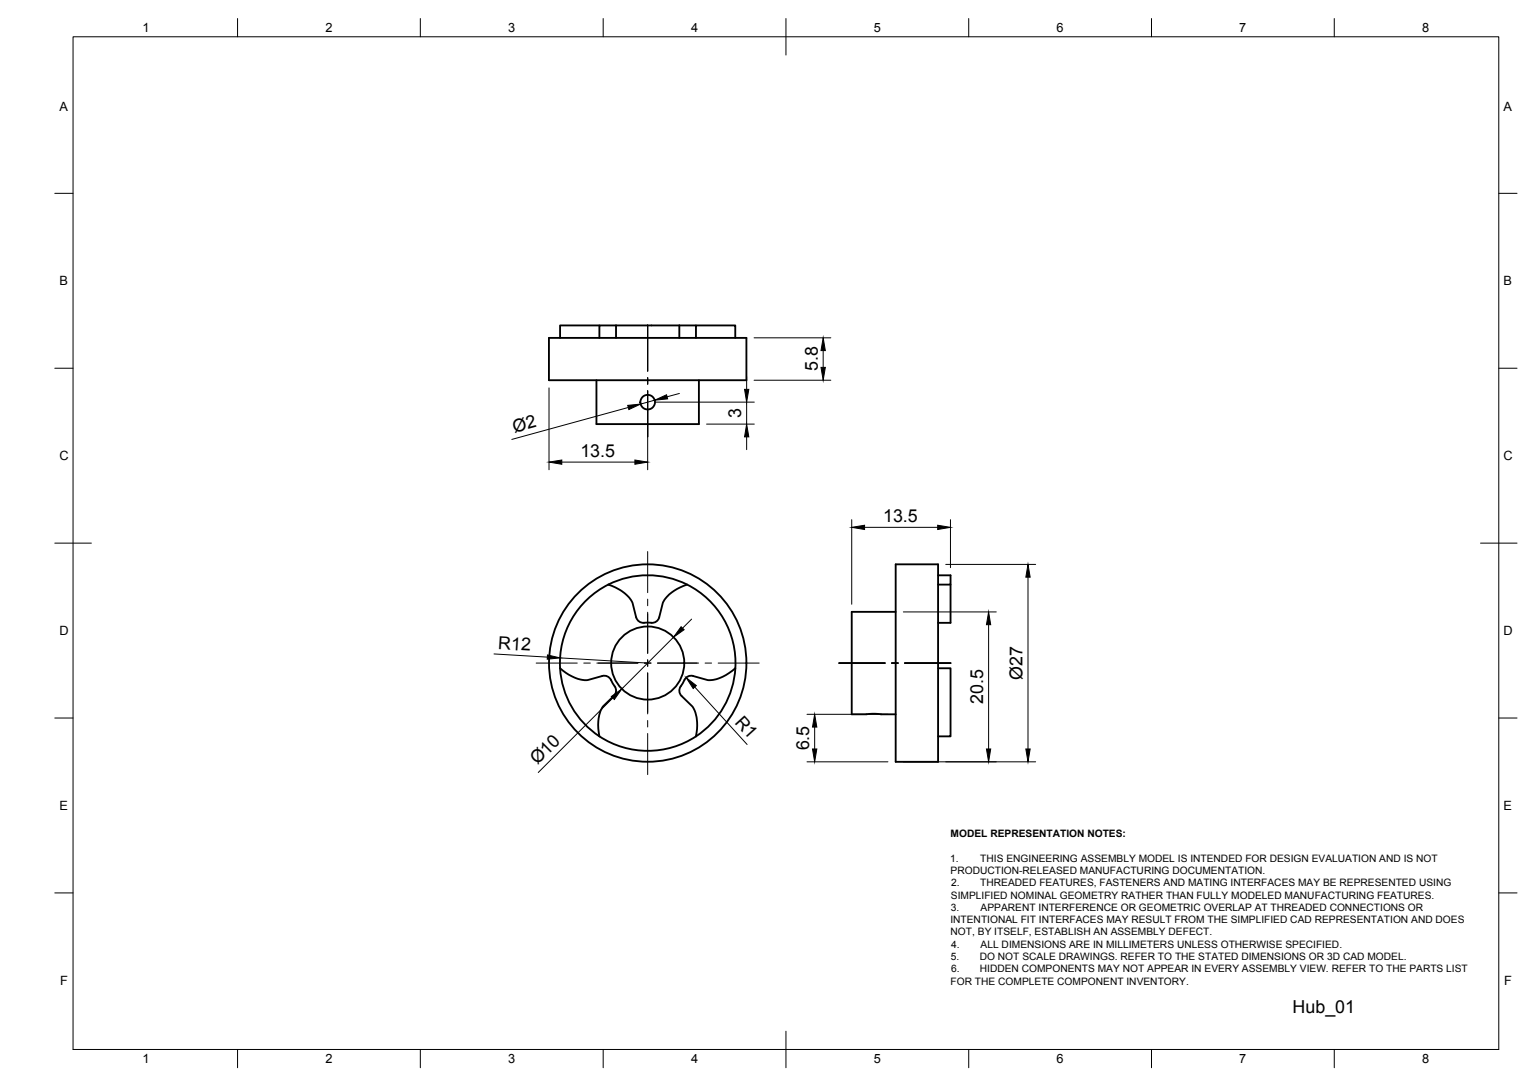
ISO-10303-21;
HEADER;
/* Generated by software containing ST-Developer
 * from STEP Tools, Inc. (www.steptools.com) 
 */

FILE_DESCRIPTION(
/* description */ (''),
/* implementation_level */ '2;1');

FILE_NAME(
/* name */ 'Hub_01.step',
/* time_stamp */ '2026-10-05T21:34:53-07:00',
/* author */ (''),
/* organization */ (''),
/* preprocessor_version */ 'ST-DEVELOPER v20.2',
/* originating_system */ 'Autodesk Translation Framework v15.15.0.0',
/* authorisation */ '');

FILE_SCHEMA (('AUTOMOTIVE_DESIGN { 1 0 10303 214 3 1 1 }'));
ENDSEC;

DATA;
#10=MECHANICAL_DESIGN_GEOMETRIC_PRESENTATION_REPRESENTATION('',(#66),#9822);
#48=SHAPE_REPRESENTATION_RELATIONSHIP('SRR','None',#9858,#57);
#57=ADVANCED_BREP_SHAPE_REPRESENTATION('',(#75),#9814);
#66=STYLED_ITEM('',(#9911),#75);
#75=MANIFOLD_SOLID_BREP('Body1',#3289);
#85=FACE_BOUND('',#514,.T.);
#86=FACE_BOUND('',#518,.T.);
#87=FACE_BOUND('',#520,.T.);
#88=FACE_BOUND('',#522,.T.);
#89=FACE_BOUND('',#525,.T.);
#123=B_SPLINE_CURVE_WITH_KNOTS('',3,(#8517,#8518,#8519,#8520,#8521,#8522,
#8523,#8524,#8525,#8526,#8527,#8528,#8529,#8530,#8531,#8532,#8533,#8534),
 .UNSPECIFIED.,.F.,.F.,(4,2,2,2,2,2,2,2,4),(0.,0.0377244205563716,0.0754488411127431,
0.113172721595804,0.150896602078865,0.188620482561925,0.226344363044986,
0.264068783601358,0.301793204157729),.UNSPECIFIED.);
#124=B_SPLINE_CURVE_WITH_KNOTS('',3,(#8535,#8536,#8537,#8538,#8539,#8540,
#8541,#8542,#8543,#8544,#8545,#8546,#8547,#8548,#8549,#8550,#8551,#8552),
 .UNSPECIFIED.,.F.,.F.,(4,2,2,2,2,2,2,2,4),(0.301793204157729,0.339517624714101,
0.377242045270472,0.414965925753533,0.452689806236594,0.490413686719655,
0.528137567202715,0.565861987759087,0.603586408315459),.UNSPECIFIED.);
#125=B_SPLINE_CURVE_WITH_KNOTS('',3,(#8568,#8569,#8570,#8571,#8572,#8573,
#8574,#8575,#8576,#8577,#8578,#8579,#8580,#8581,#8582,#8583,#8584,#8585),
 .UNSPECIFIED.,.F.,.F.,(4,2,2,2,2,2,2,2,4),(-0.302227736861757,-0.264448211272738,
-0.226668685683718,-0.188891277057298,-0.151113868430879,-0.113336459804459,
-0.0755590511780388,-0.0377795255890194,0.),.UNSPECIFIED.);
#126=B_SPLINE_CURVE_WITH_KNOTS('',3,(#8650,#8651,#8652,#8653,#8654,#8655,
#8656,#8657,#8658,#8659),.UNSPECIFIED.,.F.,.F.,(4,2,2,2,4),(-1.69587030996743,
-0.72373117051105,-0.441822634822492,-0.252830368895713,0.),
 .UNSPECIFIED.);
#127=B_SPLINE_CURVE_WITH_KNOTS('',3,(#8670,#8671,#8672,#8673,#8674,#8675,
#8676,#8677,#8678,#8679),.UNSPECIFIED.,.F.,.F.,(4,2,2,2,4),(-0.142515337540036,
-0.116550796137795,-0.0827833358078941,-0.0239794870259568,0.),
 .UNSPECIFIED.);
#128=B_SPLINE_CURVE_WITH_KNOTS('',3,(#8681,#8682,#8683,#8684,#8685,#8686,
#8687,#8688,#8689,#8690),.UNSPECIFIED.,.F.,.F.,(4,2,2,2,4),(-1.69587031141743,
-0.723731170975569,-0.441822635061051,-0.252830368989318,0.),
 .UNSPECIFIED.);
#129=B_SPLINE_CURVE_WITH_KNOTS('',3,(#8701,#8702,#8703,#8704,#8705,#8706,
#8707,#8708,#8709,#8710),.UNSPECIFIED.,.F.,.F.,(4,2,2,2,4),(-0.142515337583282,
-0.116550796158019,-0.0827833358058086,-0.0239794870257561,0.),
 .UNSPECIFIED.);
#130=B_SPLINE_CURVE_WITH_KNOTS('',3,(#8712,#8713,#8714,#8715,#8716,#8717,
#8718,#8719,#8720,#8721),.UNSPECIFIED.,.F.,.F.,(4,2,2,2,4),(-1.69587031053129,
-0.72373117069956,-0.441822634924292,-0.252830368936358,0.),
 .UNSPECIFIED.);
#131=B_SPLINE_CURVE_WITH_KNOTS('',3,(#8732,#8733,#8734,#8735,#8736,#8737,
#8738,#8739,#8740,#8741),.UNSPECIFIED.,.F.,.F.,(4,2,2,2,4),(-0.142515337525874,
-0.116550796129695,-0.0827833358062311,-0.0239794870259187,0.),
 .UNSPECIFIED.);
#132=B_SPLINE_CURVE_WITH_KNOTS('',3,(#8788,#8789,#8790,#8791,#8792,#8793,
#8794,#8795,#8796,#8797),.UNSPECIFIED.,.F.,.F.,(4,2,2,2,4),(-0.142515337540036,
-0.116550796137795,-0.0827833358078941,-0.0239794870259568,0.),
 .UNSPECIFIED.);
#133=B_SPLINE_CURVE_WITH_KNOTS('',3,(#8819,#8820,#8821,#8822,#8823,#8824,
#8825,#8826,#8827,#8828),.UNSPECIFIED.,.F.,.F.,(4,2,2,2,4),(-1.69587030996743,
-0.72373117051105,-0.441822634822492,-0.252830368895713,0.),
 .UNSPECIFIED.);
#134=B_SPLINE_CURVE_WITH_KNOTS('',3,(#8871,#8872,#8873,#8874,#8875,#8876,
#8877,#8878,#8879,#8880),.UNSPECIFIED.,.F.,.F.,(4,2,2,2,4),(-0.142515337583282,
-0.116550796158019,-0.0827833358058086,-0.0239794870257561,0.),
 .UNSPECIFIED.);
#135=B_SPLINE_CURVE_WITH_KNOTS('',3,(#8902,#8903,#8904,#8905,#8906,#8907,
#8908,#8909,#8910,#8911),.UNSPECIFIED.,.F.,.F.,(4,2,2,2,4),(-1.69587031141743,
-0.723731170975569,-0.441822635061051,-0.252830368989318,0.),
 .UNSPECIFIED.);
#136=B_SPLINE_CURVE_WITH_KNOTS('',3,(#8955,#8956,#8957,#8958,#8959,#8960,
#8961,#8962,#8963,#8964),.UNSPECIFIED.,.F.,.F.,(4,2,2,2,4),(-0.142515337525874,
-0.116550796129695,-0.0827833358062311,-0.0239794870259187,0.),
 .UNSPECIFIED.);
#137=B_SPLINE_CURVE_WITH_KNOTS('',3,(#8991,#8992,#8993,#8994,#8995,#8996,
#8997,#8998,#8999,#9000),.UNSPECIFIED.,.F.,.F.,(4,2,2,2,4),(-1.69587031053129,
-0.72373117069956,-0.441822634924292,-0.252830368936358,0.),
 .UNSPECIFIED.);
#169=B_SPLINE_SURFACE_WITH_KNOTS('',3,1,((#8768,#8769),(#8770,#8771),(#8772,
#8773),(#8774,#8775),(#8776,#8777),(#8778,#8779),(#8780,#8781),(#8782,#8783),
(#8784,#8785),(#8786,#8787)),.UNSPECIFIED.,.F.,.F.,.F.,(4,2,2,2,4),(2,2),
(-0.142515337540036,-0.116550796137795,-0.0827833358078941,-0.0239794870259568,
0.),(0.,0.78),.UNSPECIFIED.);
#170=B_SPLINE_SURFACE_WITH_KNOTS('',3,1,((#8798,#8799),(#8800,#8801),(#8802,
#8803),(#8804,#8805),(#8806,#8807),(#8808,#8809),(#8810,#8811),(#8812,#8813),
(#8814,#8815),(#8816,#8817)),.UNSPECIFIED.,.F.,.F.,.F.,(4,2,2,2,4),(2,2),
(-1.69587030996743,-0.72373117051105,-0.441822634822492,-0.252830368895713,
0.),(0.,0.78),.UNSPECIFIED.);
#171=B_SPLINE_SURFACE_WITH_KNOTS('',3,1,((#8851,#8852),(#8853,#8854),(#8855,
#8856),(#8857,#8858),(#8859,#8860),(#8861,#8862),(#8863,#8864),(#8865,#8866),
(#8867,#8868),(#8869,#8870)),.UNSPECIFIED.,.F.,.F.,.F.,(4,2,2,2,4),(2,2),
(-0.142515337583282,-0.116550796158019,-0.0827833358058086,-0.0239794870257561,
0.),(0.,0.78),.UNSPECIFIED.);
#172=B_SPLINE_SURFACE_WITH_KNOTS('',3,1,((#8881,#8882),(#8883,#8884),(#8885,
#8886),(#8887,#8888),(#8889,#8890),(#8891,#8892),(#8893,#8894),(#8895,#8896),
(#8897,#8898),(#8899,#8900)),.UNSPECIFIED.,.F.,.F.,.F.,(4,2,2,2,4),(2,2),
(-1.69587031141743,-0.723731170975569,-0.441822635061051,-0.252830368989318,
0.),(0.,0.78),.UNSPECIFIED.);
#173=B_SPLINE_SURFACE_WITH_KNOTS('',3,1,((#8934,#8935),(#8936,#8937),(#8938,
#8939),(#8940,#8941),(#8942,#8943),(#8944,#8945),(#8946,#8947),(#8948,#8949),
(#8950,#8951),(#8952,#8953)),.UNSPECIFIED.,.F.,.F.,.F.,(4,2,2,2,4),(2,2),
(-0.142515337525874,-0.116550796129695,-0.0827833358062311,-0.0239794870259187,
0.),(0.,0.78),.UNSPECIFIED.);
#174=B_SPLINE_SURFACE_WITH_KNOTS('',3,1,((#8970,#8971),(#8972,#8973),(#8974,
#8975),(#8976,#8977),(#8978,#8979),(#8980,#8981),(#8982,#8983),(#8984,#8985),
(#8986,#8987),(#8988,#8989)),.UNSPECIFIED.,.F.,.F.,.F.,(4,2,2,2,4),(2,2),
(-1.69587031053129,-0.72373117069956,-0.441822634924292,-0.252830368936358,
0.),(0.,0.78),.UNSPECIFIED.);
#195=PLANE('',#3492);
#196=PLANE('',#3494);
#197=PLANE('',#3496);
#198=PLANE('',#3497);
#199=PLANE('',#3511);
#200=PLANE('',#3520);
#201=PLANE('',#3533);
#202=PLANE('',#3536);
#203=PLANE('',#3541);
#204=PLANE('',#3542);
#205=PLANE('',#3545);
#206=PLANE('',#3550);
#207=PLANE('',#3551);
#208=PLANE('',#3554);
#209=PLANE('',#3559);
#210=PLANE('',#3562);
#211=PLANE('',#3565);
#316=FACE_OUTER_BOUND('',#503,.T.);
#317=FACE_OUTER_BOUND('',#504,.T.);
#318=FACE_OUTER_BOUND('',#505,.T.);
#319=FACE_OUTER_BOUND('',#506,.T.);
#320=FACE_OUTER_BOUND('',#507,.T.);
#321=FACE_OUTER_BOUND('',#508,.T.);
#322=FACE_OUTER_BOUND('',#509,.T.);
#323=FACE_OUTER_BOUND('',#510,.T.);
#324=FACE_OUTER_BOUND('',#511,.T.);
#325=FACE_OUTER_BOUND('',#512,.T.);
#326=FACE_OUTER_BOUND('',#513,.T.);
#327=FACE_OUTER_BOUND('',#515,.T.);
#328=FACE_OUTER_BOUND('',#516,.T.);
#329=FACE_OUTER_BOUND('',#517,.T.);
#330=FACE_OUTER_BOUND('',#519,.T.);
#331=FACE_OUTER_BOUND('',#521,.T.);
#332=FACE_OUTER_BOUND('',#523,.T.);
#333=FACE_OUTER_BOUND('',#524,.T.);
#334=FACE_OUTER_BOUND('',#526,.T.);
#335=FACE_OUTER_BOUND('',#527,.T.);
#336=FACE_OUTER_BOUND('',#528,.T.);
#337=FACE_OUTER_BOUND('',#529,.T.);
#338=FACE_OUTER_BOUND('',#530,.T.);
#339=FACE_OUTER_BOUND('',#531,.T.);
#340=FACE_OUTER_BOUND('',#532,.T.);
#341=FACE_OUTER_BOUND('',#533,.T.);
#342=FACE_OUTER_BOUND('',#534,.T.);
#343=FACE_OUTER_BOUND('',#535,.T.);
#344=FACE_OUTER_BOUND('',#536,.T.);
#345=FACE_OUTER_BOUND('',#537,.T.);
#346=FACE_OUTER_BOUND('',#538,.T.);
#347=FACE_OUTER_BOUND('',#539,.T.);
#348=FACE_OUTER_BOUND('',#540,.T.);
#349=FACE_OUTER_BOUND('',#541,.T.);
#350=FACE_OUTER_BOUND('',#542,.T.);
#351=FACE_OUTER_BOUND('',#543,.T.);
#352=FACE_OUTER_BOUND('',#544,.T.);
#353=FACE_OUTER_BOUND('',#545,.T.);
#354=FACE_OUTER_BOUND('',#546,.T.);
#355=FACE_OUTER_BOUND('',#547,.T.);
#356=FACE_OUTER_BOUND('',#548,.T.);
#357=FACE_OUTER_BOUND('',#549,.T.);
#358=FACE_OUTER_BOUND('',#550,.T.);
#503=EDGE_LOOP('',(#2386,#2387,#2388,#2389,#2390,#2391));
#504=EDGE_LOOP('',(#2392,#2393,#2394,#2395));
#505=EDGE_LOOP('',(#2396,#2397,#2398,#2399));
#506=EDGE_LOOP('',(#2400,#2401,#2402,#2403));
#507=EDGE_LOOP('',(#2404,#2405,#2406,#2407,#2408));
#508=EDGE_LOOP('',(#2409,#2410,#2411,#2412,#2413));
#509=EDGE_LOOP('',(#2414,#2415,#2416,#2417,#2418,#2419,#2420,#2421));
#510=EDGE_LOOP('',(#2422,#2423,#2424,#2425));
#511=EDGE_LOOP('',(#2426,#2427,#2428,#2429));
#512=EDGE_LOOP('',(#2430,#2431,#2432,#2433));
#513=EDGE_LOOP('',(#2434));
#514=EDGE_LOOP('',(#2435,#2436,#2437,#2438,#2439,#2440));
#515=EDGE_LOOP('',(#2441,#2442,#2443,#2444));
#516=EDGE_LOOP('',(#2445,#2446,#2447,#2448));
#517=EDGE_LOOP('',(#2449,#2450,#2451,#2452,#2453,#2454,#2455,#2456,#2457,
#2458,#2459,#2460,#2461,#2462,#2463,#2464,#2465,#2466,#2467,#2468,#2469,
#2470,#2471,#2472));
#518=EDGE_LOOP('',(#2473));
#519=EDGE_LOOP('',(#2474,#2475,#2476,#2477));
#520=EDGE_LOOP('',(#2478,#2479));
#521=EDGE_LOOP('',(#2480));
#522=EDGE_LOOP('',(#2481,#2482,#2483,#2484,#2485));
#523=EDGE_LOOP('',(#2486,#2487,#2488,#2489));
#524=EDGE_LOOP('',(#2490));
#525=EDGE_LOOP('',(#2491));
#526=EDGE_LOOP('',(#2492,#2493,#2494,#2495));
#527=EDGE_LOOP('',(#2496,#2497,#2498,#2499));
#528=EDGE_LOOP('',(#2500,#2501,#2502,#2503));
#529=EDGE_LOOP('',(#2504,#2505,#2506,#2507,#2508));
#530=EDGE_LOOP('',(#2509,#2510,#2511,#2512,#2513));
#531=EDGE_LOOP('',(#2514,#2515,#2516,#2517));
#532=EDGE_LOOP('',(#2518,#2519,#2520,#2521));
#533=EDGE_LOOP('',(#2522,#2523,#2524,#2525,#2526,#2527,#2528,#2529));
#534=EDGE_LOOP('',(#2530,#2531,#2532,#2533));
#535=EDGE_LOOP('',(#2534,#2535,#2536,#2537));
#536=EDGE_LOOP('',(#2538,#2539,#2540,#2541));
#537=EDGE_LOOP('',(#2542,#2543,#2544,#2545,#2546));
#538=EDGE_LOOP('',(#2547,#2548,#2549,#2550,#2551));
#539=EDGE_LOOP('',(#2552,#2553,#2554,#2555));
#540=EDGE_LOOP('',(#2556,#2557,#2558,#2559));
#541=EDGE_LOOP('',(#2560,#2561,#2562,#2563,#2564,#2565,#2566,#2567));
#542=EDGE_LOOP('',(#2568,#2569,#2570,#2571));
#543=EDGE_LOOP('',(#2572,#2573,#2574,#2575));
#544=EDGE_LOOP('',(#2576,#2577,#2578,#2579));
#545=EDGE_LOOP('',(#2580,#2581,#2582,#2583,#2584));
#546=EDGE_LOOP('',(#2585,#2586,#2587,#2588));
#547=EDGE_LOOP('',(#2589,#2590,#2591,#2592,#2593));
#548=EDGE_LOOP('',(#2594,#2595,#2596,#2597));
#549=EDGE_LOOP('',(#2598,#2599,#2600,#2601));
#550=EDGE_LOOP('',(#2602,#2603,#2604,#2605,#2606,#2607,#2608,#2609));
#724=LINE('',#8515,#983);
#725=LINE('',#8555,#984);
#726=LINE('',#8558,#985);
#727=LINE('',#8561,#986);
#728=LINE('',#8563,#987);
#729=LINE('',#8564,#988);
#730=LINE('',#8586,#989);
#731=LINE('',#8587,#990);
#732=LINE('',#8590,#991);
#733=LINE('',#8591,#992);
#734=LINE('',#8594,#993);
#735=LINE('',#8595,#994);
#736=LINE('',#8600,#995);
#737=LINE('',#8606,#996);
#738=LINE('',#8610,#997);
#739=LINE('',#8615,#998);
#740=LINE('',#8619,#999);
#741=LINE('',#8624,#1000);
#742=LINE('',#8628,#1001);
#743=LINE('',#8638,#1002);
#744=LINE('',#8641,#1003);
#745=LINE('',#8644,#1004);
#746=LINE('',#8647,#1005);
#747=LINE('',#8661,#1006);
#748=LINE('',#8669,#1007);
#749=LINE('',#8692,#1008);
#750=LINE('',#8700,#1009);
#751=LINE('',#8723,#1010);
#752=LINE('',#8731,#1011);
#753=LINE('',#8746,#1012);
#754=LINE('',#8752,#1013);
#755=LINE('',#8756,#1014);
#756=LINE('',#8759,#1015);
#757=LINE('',#8763,#1016);
#758=LINE('',#8766,#1017);
#759=LINE('',#8767,#1018);
#760=LINE('',#8829,#1019);
#761=LINE('',#8832,#1020);
#762=LINE('',#8833,#1021);
#763=LINE('',#8839,#1022);
#764=LINE('',#8842,#1023);
#765=LINE('',#8846,#1024);
#766=LINE('',#8849,#1025);
#767=LINE('',#8850,#1026);
#768=LINE('',#8912,#1027);
#769=LINE('',#8915,#1028);
#770=LINE('',#8916,#1029);
#771=LINE('',#8922,#1030);
#772=LINE('',#8925,#1031);
#773=LINE('',#8929,#1032);
#774=LINE('',#8932,#1033);
#775=LINE('',#8933,#1034);
#776=LINE('',#8965,#1035);
#777=LINE('',#8969,#1036);
#778=LINE('',#9001,#1037);
#779=LINE('',#9004,#1038);
#780=LINE('',#9005,#1039);
#983=VECTOR('',#3990,1.);
#984=VECTOR('',#3993,10.);
#985=VECTOR('',#3996,10.);
#986=VECTOR('',#3999,10.);
#987=VECTOR('',#4000,10.);
#988=VECTOR('',#4001,10.);
#989=VECTOR('',#4004,10.);
#990=VECTOR('',#4005,10.);
#991=VECTOR('',#4008,10.);
#992=VECTOR('',#4009,10.);
#993=VECTOR('',#4012,10.);
#994=VECTOR('',#4013,10.);
#995=VECTOR('',#4018,5.);
#996=VECTOR('',#4025,10.);
#997=VECTOR('',#4028,10.);
#998=VECTOR('',#4033,10.);
#999=VECTOR('',#4036,10.);
#1000=VECTOR('',#4041,10.);
#1001=VECTOR('',#4044,10.);
#1002=VECTOR('',#4059,10.);
#1003=VECTOR('',#4062,10.);
#1004=VECTOR('',#4065,10.);
#1005=VECTOR('',#4068,10.);
#1006=VECTOR('',#4071,10.);
#1007=VECTOR('',#4078,10.);
#1008=VECTOR('',#4079,10.);
#1009=VECTOR('',#4086,10.);
#1010=VECTOR('',#4087,10.);
#1011=VECTOR('',#4094,10.);
#1012=VECTOR('',#4099,7.);
#1013=VECTOR('',#4108,13.5);
#1014=VECTOR('',#4113,10.);
#1015=VECTOR('',#4116,10.);
#1016=VECTOR('',#4121,10.);
#1017=VECTOR('',#4124,10.);
#1018=VECTOR('',#4125,10.);
#1019=VECTOR('',#4126,10.);
#1020=VECTOR('',#4129,10.);
#1021=VECTOR('',#4130,10.);
#1022=VECTOR('',#4139,10.);
#1023=VECTOR('',#4142,10.);
#1024=VECTOR('',#4147,10.);
#1025=VECTOR('',#4150,10.);
#1026=VECTOR('',#4151,10.);
#1027=VECTOR('',#4152,10.);
#1028=VECTOR('',#4155,10.);
#1029=VECTOR('',#4156,10.);
#1030=VECTOR('',#4165,10.);
#1031=VECTOR('',#4168,10.);
#1032=VECTOR('',#4173,10.);
#1033=VECTOR('',#4176,10.);
#1034=VECTOR('',#4177,10.);
#1035=VECTOR('',#4178,10.);
#1036=VECTOR('',#4183,10.);
#1037=VECTOR('',#4184,10.);
#1038=VECTOR('',#4187,10.);
#1039=VECTOR('',#4188,10.);
#1219=CIRCLE('',#3490,1.);
#1220=CIRCLE('',#3491,1.);
#1221=CIRCLE('',#3493,1.);
#1222=CIRCLE('',#3499,5.);
#1223=CIRCLE('',#3500,5.);
#1224=CIRCLE('',#3501,5.);
#1225=CIRCLE('',#3503,12.);
#1226=CIRCLE('',#3504,12.);
#1227=CIRCLE('',#3506,12.);
#1228=CIRCLE('',#3507,12.);
#1229=CIRCLE('',#3509,12.);
#1230=CIRCLE('',#3510,12.);
#1231=CIRCLE('',#3512,13.5);
#1232=CIRCLE('',#3513,12.);
#1233=CIRCLE('',#3514,12.);
#1234=CIRCLE('',#3515,12.);
#1235=CIRCLE('',#3517,12.);
#1236=CIRCLE('',#3519,12.);
#1237=CIRCLE('',#3521,1.);
#1238=CIRCLE('',#3522,5.529);
#1239=CIRCLE('',#3523,1.);
#1240=CIRCLE('',#3524,1.);
#1241=CIRCLE('',#3525,5.529);
#1242=CIRCLE('',#3526,1.);
#1243=CIRCLE('',#3527,1.);
#1244=CIRCLE('',#3528,5.529);
#1245=CIRCLE('',#3529,1.);
#1246=CIRCLE('',#3531,7.);
#1247=CIRCLE('',#3532,7.);
#1248=CIRCLE('',#3535,13.5);
#1249=CIRCLE('',#3538,5.529);
#1250=CIRCLE('',#3540,1.);
#1251=CIRCLE('',#3544,1.);
#1252=CIRCLE('',#3547,5.529);
#1253=CIRCLE('',#3549,1.);
#1254=CIRCLE('',#3553,1.);
#1255=CIRCLE('',#3556,5.529);
#1256=CIRCLE('',#3558,1.);
#1257=CIRCLE('',#3561,12.);
#1258=CIRCLE('',#3564,1.);
#1417=VERTEX_POINT('',#8510);
#1418=VERTEX_POINT('',#8511);
#1419=VERTEX_POINT('',#8514);
#1420=VERTEX_POINT('',#8516);
#1421=VERTEX_POINT('',#8554);
#1422=VERTEX_POINT('',#8556);
#1423=VERTEX_POINT('',#8560);
#1424=VERTEX_POINT('',#8562);
#1425=VERTEX_POINT('',#8566);
#1426=VERTEX_POINT('',#8567);
#1427=VERTEX_POINT('',#8589);
#1428=VERTEX_POINT('',#8593);
#1429=VERTEX_POINT('',#8597);
#1430=VERTEX_POINT('',#8599);
#1431=VERTEX_POINT('',#8604);
#1432=VERTEX_POINT('',#8605);
#1433=VERTEX_POINT('',#8607);
#1434=VERTEX_POINT('',#8609);
#1435=VERTEX_POINT('',#8613);
#1436=VERTEX_POINT('',#8614);
#1437=VERTEX_POINT('',#8616);
#1438=VERTEX_POINT('',#8618);
#1439=VERTEX_POINT('',#8622);
#1440=VERTEX_POINT('',#8623);
#1441=VERTEX_POINT('',#8625);
#1442=VERTEX_POINT('',#8627);
#1443=VERTEX_POINT('',#8631);
#1444=VERTEX_POINT('',#8637);
#1445=VERTEX_POINT('',#8639);
#1446=VERTEX_POINT('',#8643);
#1447=VERTEX_POINT('',#8645);
#1448=VERTEX_POINT('',#8649);
#1449=VERTEX_POINT('',#8660);
#1450=VERTEX_POINT('',#8662);
#1451=VERTEX_POINT('',#8664);
#1452=VERTEX_POINT('',#8666);
#1453=VERTEX_POINT('',#8668);
#1454=VERTEX_POINT('',#8680);
#1455=VERTEX_POINT('',#8691);
#1456=VERTEX_POINT('',#8693);
#1457=VERTEX_POINT('',#8695);
#1458=VERTEX_POINT('',#8697);
#1459=VERTEX_POINT('',#8699);
#1460=VERTEX_POINT('',#8711);
#1461=VERTEX_POINT('',#8722);
#1462=VERTEX_POINT('',#8724);
#1463=VERTEX_POINT('',#8726);
#1464=VERTEX_POINT('',#8728);
#1465=VERTEX_POINT('',#8730);
#1466=VERTEX_POINT('',#8743);
#1467=VERTEX_POINT('',#8745);
#1468=VERTEX_POINT('',#8750);
#1469=VERTEX_POINT('',#8755);
#1470=VERTEX_POINT('',#8757);
#1471=VERTEX_POINT('',#8761);
#1472=VERTEX_POINT('',#8765);
#1473=VERTEX_POINT('',#8818);
#1474=VERTEX_POINT('',#8831);
#1475=VERTEX_POINT('',#8838);
#1476=VERTEX_POINT('',#8840);
#1477=VERTEX_POINT('',#8844);
#1478=VERTEX_POINT('',#8848);
#1479=VERTEX_POINT('',#8901);
#1480=VERTEX_POINT('',#8914);
#1481=VERTEX_POINT('',#8921);
#1482=VERTEX_POINT('',#8923);
#1483=VERTEX_POINT('',#8927);
#1484=VERTEX_POINT('',#8931);
#1485=VERTEX_POINT('',#8954);
#1486=VERTEX_POINT('',#8967);
#1487=VERTEX_POINT('',#8990);
#1488=VERTEX_POINT('',#9003);
#1772=EDGE_CURVE('',#1417,#1418,#1219,.T.);
#1773=EDGE_CURVE('',#1418,#1417,#1220,.T.);
#1774=EDGE_CURVE('',#1418,#1419,#724,.T.);
#1775=EDGE_CURVE('',#1420,#1419,#123,.T.);
#1776=EDGE_CURVE('',#1419,#1420,#124,.T.);
#1777=EDGE_CURVE('',#1421,#1417,#725,.T.);
#1778=EDGE_CURVE('',#1422,#1421,#1221,.T.);
#1779=EDGE_CURVE('',#1418,#1422,#726,.T.);
#1780=EDGE_CURVE('',#1423,#1418,#727,.T.);
#1781=EDGE_CURVE('',#1424,#1423,#728,.T.);
#1782=EDGE_CURVE('',#1417,#1424,#729,.T.);
#1783=EDGE_CURVE('',#1425,#1426,#125,.T.);
#1784=EDGE_CURVE('',#1425,#1422,#730,.T.);
#1785=EDGE_CURVE('',#1426,#1421,#731,.T.);
#1786=EDGE_CURVE('',#1426,#1427,#732,.T.);
#1787=EDGE_CURVE('',#1427,#1424,#733,.T.);
#1788=EDGE_CURVE('',#1428,#1425,#734,.T.);
#1789=EDGE_CURVE('',#1423,#1428,#735,.T.);
#1790=EDGE_CURVE('',#1429,#1429,#1222,.T.);
#1791=EDGE_CURVE('',#1429,#1430,#736,.T.);
#1792=EDGE_CURVE('',#1428,#1430,#1223,.T.);
#1793=EDGE_CURVE('',#1430,#1427,#1224,.T.);
#1794=EDGE_CURVE('',#1431,#1432,#737,.T.);
#1795=EDGE_CURVE('',#1433,#1431,#1225,.T.);
#1796=EDGE_CURVE('',#1433,#1434,#738,.T.);
#1797=EDGE_CURVE('',#1432,#1434,#1226,.T.);
#1798=EDGE_CURVE('',#1435,#1436,#739,.T.);
#1799=EDGE_CURVE('',#1437,#1436,#1227,.T.);
#1800=EDGE_CURVE('',#1438,#1437,#740,.T.);
#1801=EDGE_CURVE('',#1435,#1438,#1228,.T.);
#1802=EDGE_CURVE('',#1439,#1440,#741,.T.);
#1803=EDGE_CURVE('',#1441,#1440,#1229,.T.);
#1804=EDGE_CURVE('',#1442,#1441,#742,.T.);
#1805=EDGE_CURVE('',#1439,#1442,#1230,.T.);
#1806=EDGE_CURVE('',#1443,#1443,#1231,.T.);
#1807=EDGE_CURVE('',#1441,#1436,#1232,.T.);
#1808=EDGE_CURVE('',#1432,#1440,#1233,.T.);
#1809=EDGE_CURVE('',#1437,#1434,#1234,.T.);
#1810=EDGE_CURVE('',#1436,#1444,#743,.T.);
#1811=EDGE_CURVE('',#1445,#1444,#1235,.T.);
#1812=EDGE_CURVE('',#1441,#1445,#744,.T.);
#1813=EDGE_CURVE('',#1434,#1446,#745,.T.);
#1814=EDGE_CURVE('',#1447,#1446,#1236,.T.);
#1815=EDGE_CURVE('',#1437,#1447,#746,.T.);
#1816=EDGE_CURVE('',#1448,#1442,#126,.T.);
#1817=EDGE_CURVE('',#1449,#1448,#747,.T.);
#1818=EDGE_CURVE('',#1449,#1450,#1237,.T.);
#1819=EDGE_CURVE('',#1451,#1450,#1238,.T.);
#1820=EDGE_CURVE('',#1451,#1452,#1239,.T.);
#1821=EDGE_CURVE('',#1453,#1452,#748,.T.);
#1822=EDGE_CURVE('',#1435,#1453,#127,.T.);
#1823=EDGE_CURVE('',#1454,#1438,#128,.T.);
#1824=EDGE_CURVE('',#1455,#1454,#749,.T.);
#1825=EDGE_CURVE('',#1455,#1456,#1240,.T.);
#1826=EDGE_CURVE('',#1457,#1456,#1241,.T.);
#1827=EDGE_CURVE('',#1457,#1458,#1242,.T.);
#1828=EDGE_CURVE('',#1459,#1458,#750,.T.);
#1829=EDGE_CURVE('',#1433,#1459,#129,.T.);
#1830=EDGE_CURVE('',#1460,#1431,#130,.T.);
#1831=EDGE_CURVE('',#1461,#1460,#751,.T.);
#1832=EDGE_CURVE('',#1461,#1462,#1243,.T.);
#1833=EDGE_CURVE('',#1463,#1462,#1244,.T.);
#1834=EDGE_CURVE('',#1463,#1464,#1245,.T.);
#1835=EDGE_CURVE('',#1465,#1464,#752,.T.);
#1836=EDGE_CURVE('',#1439,#1465,#131,.T.);
#1837=EDGE_CURVE('',#1466,#1466,#1246,.F.);
#1838=EDGE_CURVE('',#1466,#1467,#753,.T.);
#1839=EDGE_CURVE('',#1467,#1467,#1247,.T.);
#1840=EDGE_CURVE('',#1468,#1468,#1248,.T.);
#1841=EDGE_CURVE('',#1468,#1443,#754,.T.);
#1842=EDGE_CURVE('',#1450,#1469,#755,.T.);
#1843=EDGE_CURVE('',#1470,#1469,#1249,.T.);
#1844=EDGE_CURVE('',#1451,#1470,#756,.T.);
#1845=EDGE_CURVE('',#1471,#1470,#1250,.T.);
#1846=EDGE_CURVE('',#1452,#1471,#757,.T.);
#1847=EDGE_CURVE('',#1472,#1471,#758,.T.);
#1848=EDGE_CURVE('',#1453,#1472,#759,.T.);
#1849=EDGE_CURVE('',#1444,#1472,#132,.T.);
#1850=EDGE_CURVE('',#1473,#1445,#133,.T.);
#1851=EDGE_CURVE('',#1448,#1473,#760,.T.);
#1852=EDGE_CURVE('',#1474,#1473,#761,.T.);
#1853=EDGE_CURVE('',#1449,#1474,#762,.T.);
#1854=EDGE_CURVE('',#1469,#1474,#1251,.T.);
#1855=EDGE_CURVE('',#1456,#1475,#763,.T.);
#1856=EDGE_CURVE('',#1476,#1475,#1252,.T.);
#1857=EDGE_CURVE('',#1457,#1476,#764,.T.);
#1858=EDGE_CURVE('',#1477,#1476,#1253,.T.);
#1859=EDGE_CURVE('',#1458,#1477,#765,.T.);
#1860=EDGE_CURVE('',#1478,#1477,#766,.T.);
#1861=EDGE_CURVE('',#1459,#1478,#767,.T.);
#1862=EDGE_CURVE('',#1446,#1478,#134,.T.);
#1863=EDGE_CURVE('',#1479,#1447,#135,.T.);
#1864=EDGE_CURVE('',#1454,#1479,#768,.T.);
#1865=EDGE_CURVE('',#1480,#1479,#769,.T.);
#1866=EDGE_CURVE('',#1455,#1480,#770,.T.);
#1867=EDGE_CURVE('',#1475,#1480,#1254,.T.);
#1868=EDGE_CURVE('',#1462,#1481,#771,.T.);
#1869=EDGE_CURVE('',#1482,#1481,#1255,.T.);
#1870=EDGE_CURVE('',#1463,#1482,#772,.T.);
#1871=EDGE_CURVE('',#1483,#1482,#1256,.T.);
#1872=EDGE_CURVE('',#1464,#1483,#773,.T.);
#1873=EDGE_CURVE('',#1484,#1483,#774,.T.);
#1874=EDGE_CURVE('',#1465,#1484,#775,.T.);
#1875=EDGE_CURVE('',#1485,#1484,#136,.T.);
#1876=EDGE_CURVE('',#1440,#1485,#776,.T.);
#1877=EDGE_CURVE('',#1486,#1485,#1257,.T.);
#1878=EDGE_CURVE('',#1432,#1486,#777,.T.);
#1879=EDGE_CURVE('',#1487,#1486,#137,.T.);
#1880=EDGE_CURVE('',#1460,#1487,#778,.T.);
#1881=EDGE_CURVE('',#1488,#1487,#779,.T.);
#1882=EDGE_CURVE('',#1461,#1488,#780,.T.);
#1883=EDGE_CURVE('',#1481,#1488,#1258,.T.);
#2386=ORIENTED_EDGE('',*,*,#1772,.F.);
#2387=ORIENTED_EDGE('',*,*,#1773,.F.);
#2388=ORIENTED_EDGE('',*,*,#1774,.T.);
#2389=ORIENTED_EDGE('',*,*,#1775,.F.);
#2390=ORIENTED_EDGE('',*,*,#1776,.F.);
#2391=ORIENTED_EDGE('',*,*,#1774,.F.);
#2392=ORIENTED_EDGE('',*,*,#1773,.T.);
#2393=ORIENTED_EDGE('',*,*,#1777,.F.);
#2394=ORIENTED_EDGE('',*,*,#1778,.F.);
#2395=ORIENTED_EDGE('',*,*,#1779,.F.);
#2396=ORIENTED_EDGE('',*,*,#1772,.T.);
#2397=ORIENTED_EDGE('',*,*,#1780,.F.);
#2398=ORIENTED_EDGE('',*,*,#1781,.F.);
#2399=ORIENTED_EDGE('',*,*,#1782,.F.);
#2400=ORIENTED_EDGE('',*,*,#1783,.F.);
#2401=ORIENTED_EDGE('',*,*,#1784,.T.);
#2402=ORIENTED_EDGE('',*,*,#1778,.T.);
#2403=ORIENTED_EDGE('',*,*,#1785,.F.);
#2404=ORIENTED_EDGE('',*,*,#1786,.F.);
#2405=ORIENTED_EDGE('',*,*,#1785,.T.);
#2406=ORIENTED_EDGE('',*,*,#1777,.T.);
#2407=ORIENTED_EDGE('',*,*,#1782,.T.);
#2408=ORIENTED_EDGE('',*,*,#1787,.F.);
#2409=ORIENTED_EDGE('',*,*,#1788,.F.);
#2410=ORIENTED_EDGE('',*,*,#1789,.F.);
#2411=ORIENTED_EDGE('',*,*,#1780,.T.);
#2412=ORIENTED_EDGE('',*,*,#1779,.T.);
#2413=ORIENTED_EDGE('',*,*,#1784,.F.);
#2414=ORIENTED_EDGE('',*,*,#1790,.T.);
#2415=ORIENTED_EDGE('',*,*,#1791,.T.);
#2416=ORIENTED_EDGE('',*,*,#1792,.F.);
#2417=ORIENTED_EDGE('',*,*,#1788,.T.);
#2418=ORIENTED_EDGE('',*,*,#1783,.T.);
#2419=ORIENTED_EDGE('',*,*,#1786,.T.);
#2420=ORIENTED_EDGE('',*,*,#1793,.F.);
#2421=ORIENTED_EDGE('',*,*,#1791,.F.);
#2422=ORIENTED_EDGE('',*,*,#1794,.F.);
#2423=ORIENTED_EDGE('',*,*,#1795,.F.);
#2424=ORIENTED_EDGE('',*,*,#1796,.T.);
#2425=ORIENTED_EDGE('',*,*,#1797,.F.);
#2426=ORIENTED_EDGE('',*,*,#1798,.T.);
#2427=ORIENTED_EDGE('',*,*,#1799,.F.);
#2428=ORIENTED_EDGE('',*,*,#1800,.F.);
#2429=ORIENTED_EDGE('',*,*,#1801,.F.);
#2430=ORIENTED_EDGE('',*,*,#1802,.T.);
#2431=ORIENTED_EDGE('',*,*,#1803,.F.);
#2432=ORIENTED_EDGE('',*,*,#1804,.F.);
#2433=ORIENTED_EDGE('',*,*,#1805,.F.);
#2434=ORIENTED_EDGE('',*,*,#1806,.T.);
#2435=ORIENTED_EDGE('',*,*,#1807,.F.);
#2436=ORIENTED_EDGE('',*,*,#1803,.T.);
#2437=ORIENTED_EDGE('',*,*,#1808,.F.);
#2438=ORIENTED_EDGE('',*,*,#1797,.T.);
#2439=ORIENTED_EDGE('',*,*,#1809,.F.);
#2440=ORIENTED_EDGE('',*,*,#1799,.T.);
#2441=ORIENTED_EDGE('',*,*,#1807,.T.);
#2442=ORIENTED_EDGE('',*,*,#1810,.T.);
#2443=ORIENTED_EDGE('',*,*,#1811,.F.);
#2444=ORIENTED_EDGE('',*,*,#1812,.F.);
#2445=ORIENTED_EDGE('',*,*,#1809,.T.);
#2446=ORIENTED_EDGE('',*,*,#1813,.T.);
#2447=ORIENTED_EDGE('',*,*,#1814,.F.);
#2448=ORIENTED_EDGE('',*,*,#1815,.F.);
#2449=ORIENTED_EDGE('',*,*,#1805,.T.);
#2450=ORIENTED_EDGE('',*,*,#1816,.F.);
#2451=ORIENTED_EDGE('',*,*,#1817,.F.);
#2452=ORIENTED_EDGE('',*,*,#1818,.T.);
#2453=ORIENTED_EDGE('',*,*,#1819,.F.);
#2454=ORIENTED_EDGE('',*,*,#1820,.T.);
#2455=ORIENTED_EDGE('',*,*,#1821,.F.);
#2456=ORIENTED_EDGE('',*,*,#1822,.F.);
#2457=ORIENTED_EDGE('',*,*,#1801,.T.);
#2458=ORIENTED_EDGE('',*,*,#1823,.F.);
#2459=ORIENTED_EDGE('',*,*,#1824,.F.);
#2460=ORIENTED_EDGE('',*,*,#1825,.T.);
#2461=ORIENTED_EDGE('',*,*,#1826,.F.);
#2462=ORIENTED_EDGE('',*,*,#1827,.T.);
#2463=ORIENTED_EDGE('',*,*,#1828,.F.);
#2464=ORIENTED_EDGE('',*,*,#1829,.F.);
#2465=ORIENTED_EDGE('',*,*,#1795,.T.);
#2466=ORIENTED_EDGE('',*,*,#1830,.F.);
#2467=ORIENTED_EDGE('',*,*,#1831,.F.);
#2468=ORIENTED_EDGE('',*,*,#1832,.T.);
#2469=ORIENTED_EDGE('',*,*,#1833,.F.);
#2470=ORIENTED_EDGE('',*,*,#1834,.T.);
#2471=ORIENTED_EDGE('',*,*,#1835,.F.);
#2472=ORIENTED_EDGE('',*,*,#1836,.F.);
#2473=ORIENTED_EDGE('',*,*,#1790,.F.);
#2474=ORIENTED_EDGE('',*,*,#1837,.F.);
#2475=ORIENTED_EDGE('',*,*,#1838,.T.);
#2476=ORIENTED_EDGE('',*,*,#1839,.F.);
#2477=ORIENTED_EDGE('',*,*,#1838,.F.);
#2478=ORIENTED_EDGE('',*,*,#1775,.T.);
#2479=ORIENTED_EDGE('',*,*,#1776,.T.);
#2480=ORIENTED_EDGE('',*,*,#1837,.T.);
#2481=ORIENTED_EDGE('',*,*,#1789,.T.);
#2482=ORIENTED_EDGE('',*,*,#1792,.T.);
#2483=ORIENTED_EDGE('',*,*,#1793,.T.);
#2484=ORIENTED_EDGE('',*,*,#1787,.T.);
#2485=ORIENTED_EDGE('',*,*,#1781,.T.);
#2486=ORIENTED_EDGE('',*,*,#1840,.F.);
#2487=ORIENTED_EDGE('',*,*,#1841,.T.);
#2488=ORIENTED_EDGE('',*,*,#1806,.F.);
#2489=ORIENTED_EDGE('',*,*,#1841,.F.);
#2490=ORIENTED_EDGE('',*,*,#1840,.T.);
#2491=ORIENTED_EDGE('',*,*,#1839,.T.);
#2492=ORIENTED_EDGE('',*,*,#1819,.T.);
#2493=ORIENTED_EDGE('',*,*,#1842,.T.);
#2494=ORIENTED_EDGE('',*,*,#1843,.F.);
#2495=ORIENTED_EDGE('',*,*,#1844,.F.);
#2496=ORIENTED_EDGE('',*,*,#1820,.F.);
#2497=ORIENTED_EDGE('',*,*,#1844,.T.);
#2498=ORIENTED_EDGE('',*,*,#1845,.F.);
#2499=ORIENTED_EDGE('',*,*,#1846,.F.);
#2500=ORIENTED_EDGE('',*,*,#1821,.T.);
#2501=ORIENTED_EDGE('',*,*,#1846,.T.);
#2502=ORIENTED_EDGE('',*,*,#1847,.F.);
#2503=ORIENTED_EDGE('',*,*,#1848,.F.);
#2504=ORIENTED_EDGE('',*,*,#1822,.T.);
#2505=ORIENTED_EDGE('',*,*,#1848,.T.);
#2506=ORIENTED_EDGE('',*,*,#1849,.F.);
#2507=ORIENTED_EDGE('',*,*,#1810,.F.);
#2508=ORIENTED_EDGE('',*,*,#1798,.F.);
#2509=ORIENTED_EDGE('',*,*,#1816,.T.);
#2510=ORIENTED_EDGE('',*,*,#1804,.T.);
#2511=ORIENTED_EDGE('',*,*,#1812,.T.);
#2512=ORIENTED_EDGE('',*,*,#1850,.F.);
#2513=ORIENTED_EDGE('',*,*,#1851,.F.);
#2514=ORIENTED_EDGE('',*,*,#1817,.T.);
#2515=ORIENTED_EDGE('',*,*,#1851,.T.);
#2516=ORIENTED_EDGE('',*,*,#1852,.F.);
#2517=ORIENTED_EDGE('',*,*,#1853,.F.);
#2518=ORIENTED_EDGE('',*,*,#1818,.F.);
#2519=ORIENTED_EDGE('',*,*,#1853,.T.);
#2520=ORIENTED_EDGE('',*,*,#1854,.F.);
#2521=ORIENTED_EDGE('',*,*,#1842,.F.);
#2522=ORIENTED_EDGE('',*,*,#1854,.T.);
#2523=ORIENTED_EDGE('',*,*,#1852,.T.);
#2524=ORIENTED_EDGE('',*,*,#1850,.T.);
#2525=ORIENTED_EDGE('',*,*,#1811,.T.);
#2526=ORIENTED_EDGE('',*,*,#1849,.T.);
#2527=ORIENTED_EDGE('',*,*,#1847,.T.);
#2528=ORIENTED_EDGE('',*,*,#1845,.T.);
#2529=ORIENTED_EDGE('',*,*,#1843,.T.);
#2530=ORIENTED_EDGE('',*,*,#1826,.T.);
#2531=ORIENTED_EDGE('',*,*,#1855,.T.);
#2532=ORIENTED_EDGE('',*,*,#1856,.F.);
#2533=ORIENTED_EDGE('',*,*,#1857,.F.);
#2534=ORIENTED_EDGE('',*,*,#1827,.F.);
#2535=ORIENTED_EDGE('',*,*,#1857,.T.);
#2536=ORIENTED_EDGE('',*,*,#1858,.F.);
#2537=ORIENTED_EDGE('',*,*,#1859,.F.);
#2538=ORIENTED_EDGE('',*,*,#1828,.T.);
#2539=ORIENTED_EDGE('',*,*,#1859,.T.);
#2540=ORIENTED_EDGE('',*,*,#1860,.F.);
#2541=ORIENTED_EDGE('',*,*,#1861,.F.);
#2542=ORIENTED_EDGE('',*,*,#1829,.T.);
#2543=ORIENTED_EDGE('',*,*,#1861,.T.);
#2544=ORIENTED_EDGE('',*,*,#1862,.F.);
#2545=ORIENTED_EDGE('',*,*,#1813,.F.);
#2546=ORIENTED_EDGE('',*,*,#1796,.F.);
#2547=ORIENTED_EDGE('',*,*,#1823,.T.);
#2548=ORIENTED_EDGE('',*,*,#1800,.T.);
#2549=ORIENTED_EDGE('',*,*,#1815,.T.);
#2550=ORIENTED_EDGE('',*,*,#1863,.F.);
#2551=ORIENTED_EDGE('',*,*,#1864,.F.);
#2552=ORIENTED_EDGE('',*,*,#1824,.T.);
#2553=ORIENTED_EDGE('',*,*,#1864,.T.);
#2554=ORIENTED_EDGE('',*,*,#1865,.F.);
#2555=ORIENTED_EDGE('',*,*,#1866,.F.);
#2556=ORIENTED_EDGE('',*,*,#1825,.F.);
#2557=ORIENTED_EDGE('',*,*,#1866,.T.);
#2558=ORIENTED_EDGE('',*,*,#1867,.F.);
#2559=ORIENTED_EDGE('',*,*,#1855,.F.);
#2560=ORIENTED_EDGE('',*,*,#1867,.T.);
#2561=ORIENTED_EDGE('',*,*,#1865,.T.);
#2562=ORIENTED_EDGE('',*,*,#1863,.T.);
#2563=ORIENTED_EDGE('',*,*,#1814,.T.);
#2564=ORIENTED_EDGE('',*,*,#1862,.T.);
#2565=ORIENTED_EDGE('',*,*,#1860,.T.);
#2566=ORIENTED_EDGE('',*,*,#1858,.T.);
#2567=ORIENTED_EDGE('',*,*,#1856,.T.);
#2568=ORIENTED_EDGE('',*,*,#1833,.T.);
#2569=ORIENTED_EDGE('',*,*,#1868,.T.);
#2570=ORIENTED_EDGE('',*,*,#1869,.F.);
#2571=ORIENTED_EDGE('',*,*,#1870,.F.);
#2572=ORIENTED_EDGE('',*,*,#1834,.F.);
#2573=ORIENTED_EDGE('',*,*,#1870,.T.);
#2574=ORIENTED_EDGE('',*,*,#1871,.F.);
#2575=ORIENTED_EDGE('',*,*,#1872,.F.);
#2576=ORIENTED_EDGE('',*,*,#1835,.T.);
#2577=ORIENTED_EDGE('',*,*,#1872,.T.);
#2578=ORIENTED_EDGE('',*,*,#1873,.F.);
#2579=ORIENTED_EDGE('',*,*,#1874,.F.);
#2580=ORIENTED_EDGE('',*,*,#1836,.T.);
#2581=ORIENTED_EDGE('',*,*,#1874,.T.);
#2582=ORIENTED_EDGE('',*,*,#1875,.F.);
#2583=ORIENTED_EDGE('',*,*,#1876,.F.);
#2584=ORIENTED_EDGE('',*,*,#1802,.F.);
#2585=ORIENTED_EDGE('',*,*,#1808,.T.);
#2586=ORIENTED_EDGE('',*,*,#1876,.T.);
#2587=ORIENTED_EDGE('',*,*,#1877,.F.);
#2588=ORIENTED_EDGE('',*,*,#1878,.F.);
#2589=ORIENTED_EDGE('',*,*,#1830,.T.);
#2590=ORIENTED_EDGE('',*,*,#1794,.T.);
#2591=ORIENTED_EDGE('',*,*,#1878,.T.);
#2592=ORIENTED_EDGE('',*,*,#1879,.F.);
#2593=ORIENTED_EDGE('',*,*,#1880,.F.);
#2594=ORIENTED_EDGE('',*,*,#1831,.T.);
#2595=ORIENTED_EDGE('',*,*,#1880,.T.);
#2596=ORIENTED_EDGE('',*,*,#1881,.F.);
#2597=ORIENTED_EDGE('',*,*,#1882,.F.);
#2598=ORIENTED_EDGE('',*,*,#1832,.F.);
#2599=ORIENTED_EDGE('',*,*,#1882,.T.);
#2600=ORIENTED_EDGE('',*,*,#1883,.F.);
#2601=ORIENTED_EDGE('',*,*,#1868,.F.);
#2602=ORIENTED_EDGE('',*,*,#1883,.T.);
#2603=ORIENTED_EDGE('',*,*,#1881,.T.);
#2604=ORIENTED_EDGE('',*,*,#1879,.T.);
#2605=ORIENTED_EDGE('',*,*,#1877,.T.);
#2606=ORIENTED_EDGE('',*,*,#1875,.T.);
#2607=ORIENTED_EDGE('',*,*,#1873,.T.);
#2608=ORIENTED_EDGE('',*,*,#1871,.T.);
#2609=ORIENTED_EDGE('',*,*,#1869,.T.);
#3051=CYLINDRICAL_SURFACE('',#3489,1.);
#3052=CYLINDRICAL_SURFACE('',#3495,1.);
#3053=CYLINDRICAL_SURFACE('',#3498,5.);
#3054=CYLINDRICAL_SURFACE('',#3502,12.);
#3055=CYLINDRICAL_SURFACE('',#3505,12.);
#3056=CYLINDRICAL_SURFACE('',#3508,12.);
#3057=CYLINDRICAL_SURFACE('',#3516,12.);
#3058=CYLINDRICAL_SURFACE('',#3518,12.);
#3059=CYLINDRICAL_SURFACE('',#3530,7.);
#3060=CYLINDRICAL_SURFACE('',#3534,13.5);
#3061=CYLINDRICAL_SURFACE('',#3537,5.529);
#3062=CYLINDRICAL_SURFACE('',#3539,1.);
#3063=CYLINDRICAL_SURFACE('',#3543,1.);
#3064=CYLINDRICAL_SURFACE('',#3546,5.529);
#3065=CYLINDRICAL_SURFACE('',#3548,1.);
#3066=CYLINDRICAL_SURFACE('',#3552,1.);
#3067=CYLINDRICAL_SURFACE('',#3555,5.529);
#3068=CYLINDRICAL_SURFACE('',#3557,1.);
#3069=CYLINDRICAL_SURFACE('',#3560,12.);
#3070=CYLINDRICAL_SURFACE('',#3563,1.);
#3154=ADVANCED_FACE('',(#316),#3051,.F.);
#3155=ADVANCED_FACE('',(#317),#195,.T.);
#3156=ADVANCED_FACE('',(#318),#196,.T.);
#3157=ADVANCED_FACE('',(#319),#3052,.F.);
#3158=ADVANCED_FACE('',(#320),#197,.F.);
#3159=ADVANCED_FACE('',(#321),#198,.F.);
#3160=ADVANCED_FACE('',(#322),#3053,.F.);
#3161=ADVANCED_FACE('',(#323),#3054,.F.);
#3162=ADVANCED_FACE('',(#324),#3055,.F.);
#3163=ADVANCED_FACE('',(#325),#3056,.F.);
#3164=ADVANCED_FACE('',(#326,#85),#199,.F.);
#3165=ADVANCED_FACE('',(#327),#3057,.T.);
#3166=ADVANCED_FACE('',(#328),#3058,.T.);
#3167=ADVANCED_FACE('',(#329,#86),#200,.F.);
#3168=ADVANCED_FACE('',(#330,#87),#3059,.T.);
#3169=ADVANCED_FACE('',(#331,#88),#201,.T.);
#3170=ADVANCED_FACE('',(#332),#3060,.T.);
#3171=ADVANCED_FACE('',(#333,#89),#202,.T.);
#3172=ADVANCED_FACE('',(#334),#3061,.F.);
#3173=ADVANCED_FACE('',(#335),#3062,.T.);
#3174=ADVANCED_FACE('',(#336),#203,.T.);
#3175=ADVANCED_FACE('',(#337),#169,.T.);
#3176=ADVANCED_FACE('',(#338),#170,.T.);
#3177=ADVANCED_FACE('',(#339),#204,.T.);
#3178=ADVANCED_FACE('',(#340),#3063,.T.);
#3179=ADVANCED_FACE('',(#341),#205,.F.);
#3180=ADVANCED_FACE('',(#342),#3064,.F.);
#3181=ADVANCED_FACE('',(#343),#3065,.T.);
#3182=ADVANCED_FACE('',(#344),#206,.T.);
#3183=ADVANCED_FACE('',(#345),#171,.T.);
#3184=ADVANCED_FACE('',(#346),#172,.T.);
#3185=ADVANCED_FACE('',(#347),#207,.T.);
#3186=ADVANCED_FACE('',(#348),#3066,.T.);
#3187=ADVANCED_FACE('',(#349),#208,.F.);
#3188=ADVANCED_FACE('',(#350),#3067,.F.);
#3189=ADVANCED_FACE('',(#351),#3068,.T.);
#3190=ADVANCED_FACE('',(#352),#209,.T.);
#3191=ADVANCED_FACE('',(#353),#173,.T.);
#3192=ADVANCED_FACE('',(#354),#3069,.T.);
#3193=ADVANCED_FACE('',(#355),#174,.T.);
#3194=ADVANCED_FACE('',(#356),#210,.T.);
#3195=ADVANCED_FACE('',(#357),#3070,.T.);
#3196=ADVANCED_FACE('',(#358),#211,.F.);
#3289=CLOSED_SHELL('',(#3154,#3155,#3156,#3157,#3158,#3159,#3160,#3161,
#3162,#3163,#3164,#3165,#3166,#3167,#3168,#3169,#3170,#3171,#3172,#3173,
#3174,#3175,#3176,#3177,#3178,#3179,#3180,#3181,#3182,#3183,#3184,#3185,
#3186,#3187,#3188,#3189,#3190,#3191,#3192,#3193,#3194,#3195,#3196));
#3488=AXIS2_PLACEMENT_3D('',#8508,#3982,#3983);
#3489=AXIS2_PLACEMENT_3D('',#8509,#3984,#3985);
#3490=AXIS2_PLACEMENT_3D('',#8512,#3986,#3987);
#3491=AXIS2_PLACEMENT_3D('',#8513,#3988,#3989);
#3492=AXIS2_PLACEMENT_3D('',#8553,#3991,#3992);
#3493=AXIS2_PLACEMENT_3D('',#8557,#3994,#3995);
#3494=AXIS2_PLACEMENT_3D('',#8559,#3997,#3998);
#3495=AXIS2_PLACEMENT_3D('',#8565,#4002,#4003);
#3496=AXIS2_PLACEMENT_3D('',#8588,#4006,#4007);
#3497=AXIS2_PLACEMENT_3D('',#8592,#4010,#4011);
#3498=AXIS2_PLACEMENT_3D('',#8596,#4014,#4015);
#3499=AXIS2_PLACEMENT_3D('',#8598,#4016,#4017);
#3500=AXIS2_PLACEMENT_3D('',#8601,#4019,#4020);
#3501=AXIS2_PLACEMENT_3D('',#8602,#4021,#4022);
#3502=AXIS2_PLACEMENT_3D('',#8603,#4023,#4024);
#3503=AXIS2_PLACEMENT_3D('',#8608,#4026,#4027);
#3504=AXIS2_PLACEMENT_3D('',#8611,#4029,#4030);
#3505=AXIS2_PLACEMENT_3D('',#8612,#4031,#4032);
#3506=AXIS2_PLACEMENT_3D('',#8617,#4034,#4035);
#3507=AXIS2_PLACEMENT_3D('',#8620,#4037,#4038);
#3508=AXIS2_PLACEMENT_3D('',#8621,#4039,#4040);
#3509=AXIS2_PLACEMENT_3D('',#8626,#4042,#4043);
#3510=AXIS2_PLACEMENT_3D('',#8629,#4045,#4046);
#3511=AXIS2_PLACEMENT_3D('',#8630,#4047,#4048);
#3512=AXIS2_PLACEMENT_3D('',#8632,#4049,#4050);
#3513=AXIS2_PLACEMENT_3D('',#8633,#4051,#4052);
#3514=AXIS2_PLACEMENT_3D('',#8634,#4053,#4054);
#3515=AXIS2_PLACEMENT_3D('',#8635,#4055,#4056);
#3516=AXIS2_PLACEMENT_3D('',#8636,#4057,#4058);
#3517=AXIS2_PLACEMENT_3D('',#8640,#4060,#4061);
#3518=AXIS2_PLACEMENT_3D('',#8642,#4063,#4064);
#3519=AXIS2_PLACEMENT_3D('',#8646,#4066,#4067);
#3520=AXIS2_PLACEMENT_3D('',#8648,#4069,#4070);
#3521=AXIS2_PLACEMENT_3D('',#8663,#4072,#4073);
#3522=AXIS2_PLACEMENT_3D('',#8665,#4074,#4075);
#3523=AXIS2_PLACEMENT_3D('',#8667,#4076,#4077);
#3524=AXIS2_PLACEMENT_3D('',#8694,#4080,#4081);
#3525=AXIS2_PLACEMENT_3D('',#8696,#4082,#4083);
#3526=AXIS2_PLACEMENT_3D('',#8698,#4084,#4085);
#3527=AXIS2_PLACEMENT_3D('',#8725,#4088,#4089);
#3528=AXIS2_PLACEMENT_3D('',#8727,#4090,#4091);
#3529=AXIS2_PLACEMENT_3D('',#8729,#4092,#4093);
#3530=AXIS2_PLACEMENT_3D('',#8742,#4095,#4096);
#3531=AXIS2_PLACEMENT_3D('',#8744,#4097,#4098);
#3532=AXIS2_PLACEMENT_3D('',#8747,#4100,#4101);
#3533=AXIS2_PLACEMENT_3D('',#8748,#4102,#4103);
#3534=AXIS2_PLACEMENT_3D('',#8749,#4104,#4105);
#3535=AXIS2_PLACEMENT_3D('',#8751,#4106,#4107);
#3536=AXIS2_PLACEMENT_3D('',#8753,#4109,#4110);
#3537=AXIS2_PLACEMENT_3D('',#8754,#4111,#4112);
#3538=AXIS2_PLACEMENT_3D('',#8758,#4114,#4115);
#3539=AXIS2_PLACEMENT_3D('',#8760,#4117,#4118);
#3540=AXIS2_PLACEMENT_3D('',#8762,#4119,#4120);
#3541=AXIS2_PLACEMENT_3D('',#8764,#4122,#4123);
#3542=AXIS2_PLACEMENT_3D('',#8830,#4127,#4128);
#3543=AXIS2_PLACEMENT_3D('',#8834,#4131,#4132);
#3544=AXIS2_PLACEMENT_3D('',#8835,#4133,#4134);
#3545=AXIS2_PLACEMENT_3D('',#8836,#4135,#4136);
#3546=AXIS2_PLACEMENT_3D('',#8837,#4137,#4138);
#3547=AXIS2_PLACEMENT_3D('',#8841,#4140,#4141);
#3548=AXIS2_PLACEMENT_3D('',#8843,#4143,#4144);
#3549=AXIS2_PLACEMENT_3D('',#8845,#4145,#4146);
#3550=AXIS2_PLACEMENT_3D('',#8847,#4148,#4149);
#3551=AXIS2_PLACEMENT_3D('',#8913,#4153,#4154);
#3552=AXIS2_PLACEMENT_3D('',#8917,#4157,#4158);
#3553=AXIS2_PLACEMENT_3D('',#8918,#4159,#4160);
#3554=AXIS2_PLACEMENT_3D('',#8919,#4161,#4162);
#3555=AXIS2_PLACEMENT_3D('',#8920,#4163,#4164);
#3556=AXIS2_PLACEMENT_3D('',#8924,#4166,#4167);
#3557=AXIS2_PLACEMENT_3D('',#8926,#4169,#4170);
#3558=AXIS2_PLACEMENT_3D('',#8928,#4171,#4172);
#3559=AXIS2_PLACEMENT_3D('',#8930,#4174,#4175);
#3560=AXIS2_PLACEMENT_3D('',#8966,#4179,#4180);
#3561=AXIS2_PLACEMENT_3D('',#8968,#4181,#4182);
#3562=AXIS2_PLACEMENT_3D('',#9002,#4185,#4186);
#3563=AXIS2_PLACEMENT_3D('',#9006,#4189,#4190);
#3564=AXIS2_PLACEMENT_3D('',#9007,#4191,#4192);
#3565=AXIS2_PLACEMENT_3D('',#9008,#4193,#4194);
#3982=DIRECTION('axis',(0.,0.,1.));
#3983=DIRECTION('refdir',(1.,0.,0.));
#3984=DIRECTION('center_axis',(0.,-1.,0.));
#3985=DIRECTION('ref_axis',(1.,0.,0.));
#3986=DIRECTION('center_axis',(0.,-1.,0.));
#3987=DIRECTION('ref_axis',(1.,0.,0.));
#3988=DIRECTION('center_axis',(0.,-1.,0.));
#3989=DIRECTION('ref_axis',(1.,0.,0.));
#3990=DIRECTION('',(0.,-1.,0.));
#3991=DIRECTION('center_axis',(0.,1.,0.));
#3992=DIRECTION('ref_axis',(1.,0.,0.));
#3993=DIRECTION('',(0.,0.,1.));
#3994=DIRECTION('center_axis',(0.,-1.,0.));
#3995=DIRECTION('ref_axis',(1.,0.,0.));
#3996=DIRECTION('',(0.,0.,-1.));
#3997=DIRECTION('center_axis',(0.,1.,0.));
#3998=DIRECTION('ref_axis',(1.,0.,0.));
#3999=DIRECTION('',(0.,0.,-1.));
#4000=DIRECTION('',(-1.,0.,0.));
#4001=DIRECTION('',(0.,0.,1.));
#4002=DIRECTION('center_axis',(0.,-1.,0.));
#4003=DIRECTION('ref_axis',(1.,0.,0.));
#4004=DIRECTION('',(0.,-1.,0.));
#4005=DIRECTION('',(0.,-1.,0.));
#4006=DIRECTION('center_axis',(1.,0.,0.));
#4007=DIRECTION('ref_axis',(0.,0.,1.));
#4008=DIRECTION('',(0.,0.,1.));
#4009=DIRECTION('',(0.,-1.,0.));
#4010=DIRECTION('center_axis',(-1.,0.,0.));
#4011=DIRECTION('ref_axis',(0.,0.,-1.));
#4012=DIRECTION('',(0.,0.,-1.));
#4013=DIRECTION('',(0.,1.,0.));
#4014=DIRECTION('center_axis',(0.,0.,1.));
#4015=DIRECTION('ref_axis',(1.,0.,0.));
#4016=DIRECTION('center_axis',(0.,0.,-1.));
#4017=DIRECTION('ref_axis',(1.,0.,0.));
#4018=DIRECTION('',(0.,0.,1.));
#4019=DIRECTION('center_axis',(0.,0.,-1.));
#4020=DIRECTION('ref_axis',(-1.,0.,0.));
#4021=DIRECTION('center_axis',(0.,0.,-1.));
#4022=DIRECTION('ref_axis',(-1.,0.,0.));
#4023=DIRECTION('center_axis',(0.,0.,-1.));
#4024=DIRECTION('ref_axis',(1.,0.,0.));
#4025=DIRECTION('',(0.,0.,-1.));
#4026=DIRECTION('center_axis',(0.,0.,-1.));
#4027=DIRECTION('ref_axis',(1.,0.,0.));
#4028=DIRECTION('',(0.,0.,-1.));
#4029=DIRECTION('center_axis',(0.,0.,1.));
#4030=DIRECTION('ref_axis',(1.,0.,0.));
#4031=DIRECTION('center_axis',(0.,0.,-1.));
#4032=DIRECTION('ref_axis',(-0.866025403784439,0.5,0.));
#4033=DIRECTION('',(0.,0.,-1.));
#4034=DIRECTION('center_axis',(0.,0.,1.));
#4035=DIRECTION('ref_axis',(1.,0.,0.));
#4036=DIRECTION('',(0.,0.,-1.));
#4037=DIRECTION('center_axis',(0.,0.,-1.));
#4038=DIRECTION('ref_axis',(1.,0.,0.));
#4039=DIRECTION('center_axis',(0.,0.,-1.));
#4040=DIRECTION('ref_axis',(1.,0.,0.));
#4041=DIRECTION('',(0.,0.,-1.));
#4042=DIRECTION('center_axis',(0.,0.,1.));
#4043=DIRECTION('ref_axis',(1.,0.,0.));
#4044=DIRECTION('',(0.,0.,-1.));
#4045=DIRECTION('center_axis',(0.,0.,-1.));
#4046=DIRECTION('ref_axis',(1.,0.,0.));
#4047=DIRECTION('center_axis',(0.,0.,1.));
#4048=DIRECTION('ref_axis',(1.,0.,0.));
#4049=DIRECTION('center_axis',(0.,0.,-1.));
#4050=DIRECTION('ref_axis',(1.,0.,0.));
#4051=DIRECTION('center_axis',(0.,0.,-1.));
#4052=DIRECTION('ref_axis',(1.,0.,0.));
#4053=DIRECTION('center_axis',(0.,0.,-1.));
#4054=DIRECTION('ref_axis',(1.,0.,0.));
#4055=DIRECTION('center_axis',(0.,0.,-1.));
#4056=DIRECTION('ref_axis',(1.,0.,0.));
#4057=DIRECTION('center_axis',(0.,0.,-1.));
#4058=DIRECTION('ref_axis',(1.,0.,0.));
#4059=DIRECTION('',(0.,0.,-1.));
#4060=DIRECTION('center_axis',(0.,0.,-1.));
#4061=DIRECTION('ref_axis',(1.,0.,0.));
#4062=DIRECTION('',(0.,0.,-1.));
#4063=DIRECTION('center_axis',(0.,0.,-1.));
#4064=DIRECTION('ref_axis',(1.,0.,0.));
#4065=DIRECTION('',(0.,0.,-1.));
#4066=DIRECTION('center_axis',(0.,0.,-1.));
#4067=DIRECTION('ref_axis',(1.,0.,0.));
#4068=DIRECTION('',(0.,0.,-1.));
#4069=DIRECTION('center_axis',(0.,0.,1.));
#4070=DIRECTION('ref_axis',(1.,0.,0.));
#4071=DIRECTION('',(-0.717566844774038,-0.696489643340827,0.));
#4072=DIRECTION('center_axis',(0.,0.,1.));
#4073=DIRECTION('ref_axis',(0.696489643340827,-0.717566844774038,0.));
#4074=DIRECTION('center_axis',(0.,0.,1.));
#4075=DIRECTION('ref_axis',(-0.908768955427354,-0.417299635335902,0.));
#4076=DIRECTION('center_axis',(0.,0.,1.));
#4077=DIRECTION('ref_axis',(0.908768955427354,0.417299635335902,0.));
#4078=DIRECTION('',(0.961961146992938,0.273186294817348,0.));
#4079=DIRECTION('',(-0.2443943022189,0.969675938158175,0.));
#4080=DIRECTION('center_axis',(0.,0.,1.));
#4081=DIRECTION('ref_axis',(-0.969675938158175,-0.244394302218901,0.));
#4082=DIRECTION('center_axis',(0.,0.,1.));
#4083=DIRECTION('ref_axis',(0.0929923925228028,0.995666819238687,0.));
#4084=DIRECTION('center_axis',(0.,0.,1.));
#4085=DIRECTION('ref_axis',(-0.0929923925228032,-0.995666819238687,0.));
#4086=DIRECTION('',(-0.244394302218901,-0.969675938158175,0.));
#4087=DIRECTION('',(0.961961146992938,-0.273186294817347,0.));
#4088=DIRECTION('center_axis',(0.,0.,1.));
#4089=DIRECTION('ref_axis',(0.273186294817348,0.961961146992938,0.));
#4090=DIRECTION('center_axis',(0.,0.,1.));
#4091=DIRECTION('ref_axis',(0.81577656290455,-0.578367183902786,0.));
#4092=DIRECTION('center_axis',(0.,0.,1.));
#4093=DIRECTION('ref_axis',(-0.815776562904551,0.578367183902784,0.));
#4094=DIRECTION('',(-0.717566844774037,0.696489643340828,0.));
#4095=DIRECTION('center_axis',(0.,0.,1.));
#4096=DIRECTION('ref_axis',(-1.,0.,0.));
#4097=DIRECTION('center_axis',(0.,0.,-1.));
#4098=DIRECTION('ref_axis',(-1.,0.,0.));
#4099=DIRECTION('',(0.,0.,-1.));
#4100=DIRECTION('center_axis',(0.,0.,-1.));
#4101=DIRECTION('ref_axis',(-1.,0.,0.));
#4102=DIRECTION('center_axis',(0.,0.,1.));
#4103=DIRECTION('ref_axis',(-1.,0.,0.));
#4104=DIRECTION('center_axis',(0.,0.,1.));
#4105=DIRECTION('ref_axis',(1.,0.,0.));
#4106=DIRECTION('center_axis',(0.,0.,1.));
#4107=DIRECTION('ref_axis',(1.,0.,0.));
#4108=DIRECTION('',(0.,0.,-1.));
#4109=DIRECTION('center_axis',(0.,0.,1.));
#4110=DIRECTION('ref_axis',(1.,0.,0.));
#4111=DIRECTION('center_axis',(0.,0.,-1.));
#4112=DIRECTION('ref_axis',(-0.908768955427354,-0.417299635335902,0.));
#4113=DIRECTION('',(0.,0.,-1.));
#4114=DIRECTION('center_axis',(0.,0.,1.));
#4115=DIRECTION('ref_axis',(-0.908768955427354,-0.417299635335902,0.));
#4116=DIRECTION('',(0.,0.,-1.));
#4117=DIRECTION('center_axis',(0.,0.,-1.));
#4118=DIRECTION('ref_axis',(0.908768955427354,0.417299635335902,0.));
#4119=DIRECTION('center_axis',(0.,0.,-1.));
#4120=DIRECTION('ref_axis',(0.908768955427354,0.417299635335902,0.));
#4121=DIRECTION('',(0.,0.,-1.));
#4122=DIRECTION('center_axis',(-0.273186294817348,0.961961146992938,0.));
#4123=DIRECTION('ref_axis',(0.961961146992938,0.273186294817348,0.));
#4124=DIRECTION('',(0.961961146992938,0.273186294817348,0.));
#4125=DIRECTION('',(0.,0.,-1.));
#4126=DIRECTION('',(0.,0.,-1.));
#4127=DIRECTION('center_axis',(0.696489643340827,-0.717566844774038,0.));
#4128=DIRECTION('ref_axis',(-0.717566844774038,-0.696489643340827,0.));
#4129=DIRECTION('',(-0.717566844774038,-0.696489643340827,0.));
#4130=DIRECTION('',(0.,0.,-1.));
#4131=DIRECTION('center_axis',(0.,0.,-1.));
#4132=DIRECTION('ref_axis',(0.696489643340827,-0.717566844774038,0.));
#4133=DIRECTION('center_axis',(0.,0.,-1.));
#4134=DIRECTION('ref_axis',(0.696489643340827,-0.717566844774038,0.));
#4135=DIRECTION('center_axis',(0.,0.,1.));
#4136=DIRECTION('ref_axis',(1.,0.,0.));
#4137=DIRECTION('center_axis',(0.,0.,-1.));
#4138=DIRECTION('ref_axis',(0.0929923925228028,0.995666819238687,0.));
#4139=DIRECTION('',(0.,0.,-1.));
#4140=DIRECTION('center_axis',(0.,0.,1.));
#4141=DIRECTION('ref_axis',(0.0929923925228028,0.995666819238687,0.));
#4142=DIRECTION('',(0.,0.,-1.));
#4143=DIRECTION('center_axis',(0.,0.,-1.));
#4144=DIRECTION('ref_axis',(-0.0929923925228032,-0.995666819238687,0.));
#4145=DIRECTION('center_axis',(0.,0.,-1.));
#4146=DIRECTION('ref_axis',(-0.0929923925228032,-0.995666819238687,0.));
#4147=DIRECTION('',(0.,0.,-1.));
#4148=DIRECTION('center_axis',(0.969675938158175,-0.244394302218901,0.));
#4149=DIRECTION('ref_axis',(-0.244394302218901,-0.969675938158175,0.));
#4150=DIRECTION('',(-0.244394302218901,-0.969675938158175,0.));
#4151=DIRECTION('',(0.,0.,-1.));
#4152=DIRECTION('',(0.,0.,-1.));
#4153=DIRECTION('center_axis',(-0.969675938158175,-0.2443943022189,0.));
#4154=DIRECTION('ref_axis',(-0.2443943022189,0.969675938158175,0.));
#4155=DIRECTION('',(-0.2443943022189,0.969675938158175,0.));
#4156=DIRECTION('',(0.,0.,-1.));
#4157=DIRECTION('center_axis',(0.,0.,-1.));
#4158=DIRECTION('ref_axis',(-0.969675938158175,-0.244394302218901,0.));
#4159=DIRECTION('center_axis',(0.,0.,-1.));
#4160=DIRECTION('ref_axis',(-0.969675938158175,-0.244394302218901,0.));
#4161=DIRECTION('center_axis',(0.,0.,1.));
#4162=DIRECTION('ref_axis',(1.,0.,0.));
#4163=DIRECTION('center_axis',(0.,0.,-1.));
#4164=DIRECTION('ref_axis',(0.81577656290455,-0.578367183902786,0.));
#4165=DIRECTION('',(0.,0.,-1.));
#4166=DIRECTION('center_axis',(0.,0.,1.));
#4167=DIRECTION('ref_axis',(0.81577656290455,-0.578367183902786,0.));
#4168=DIRECTION('',(0.,0.,-1.));
#4169=DIRECTION('center_axis',(0.,0.,-1.));
#4170=DIRECTION('ref_axis',(-0.815776562904551,0.578367183902784,0.));
#4171=DIRECTION('center_axis',(0.,0.,-1.));
#4172=DIRECTION('ref_axis',(-0.815776562904551,0.578367183902784,0.));
#4173=DIRECTION('',(0.,0.,-1.));
#4174=DIRECTION('center_axis',(-0.696489643340828,-0.717566844774037,0.));
#4175=DIRECTION('ref_axis',(-0.717566844774037,0.696489643340828,0.));
#4176=DIRECTION('',(-0.717566844774037,0.696489643340828,0.));
#4177=DIRECTION('',(0.,0.,-1.));
#4178=DIRECTION('',(0.,0.,-1.));
#4179=DIRECTION('center_axis',(0.,0.,-1.));
#4180=DIRECTION('ref_axis',(1.,0.,0.));
#4181=DIRECTION('center_axis',(0.,0.,-1.));
#4182=DIRECTION('ref_axis',(1.,0.,0.));
#4183=DIRECTION('',(0.,0.,-1.));
#4184=DIRECTION('',(0.,0.,-1.));
#4185=DIRECTION('center_axis',(0.273186294817347,0.961961146992938,0.));
#4186=DIRECTION('ref_axis',(0.961961146992938,-0.273186294817347,0.));
#4187=DIRECTION('',(0.961961146992938,-0.273186294817347,0.));
#4188=DIRECTION('',(0.,0.,-1.));
#4189=DIRECTION('center_axis',(0.,0.,-1.));
#4190=DIRECTION('ref_axis',(0.273186294817348,0.961961146992938,0.));
#4191=DIRECTION('center_axis',(0.,0.,-1.));
#4192=DIRECTION('ref_axis',(0.273186294817348,0.961961146992938,0.));
#4193=DIRECTION('center_axis',(0.,0.,1.));
#4194=DIRECTION('ref_axis',(1.,0.,0.));
#8508=CARTESIAN_POINT('',(0.,0.,0.));
#8509=CARTESIAN_POINT('Origin',(0.,-6.,9.));
#8510=CARTESIAN_POINT('',(1.,-6.,9.));
#8511=CARTESIAN_POINT('',(-1.,-6.,9.));
#8512=CARTESIAN_POINT('Origin',(0.,-6.,9.));
#8513=CARTESIAN_POINT('Origin',(0.,-6.,9.));
#8514=CARTESIAN_POINT('',(-1.,-6.92820323027551,9.));
#8515=CARTESIAN_POINT('',(-1.,-6.,9.));
#8516=CARTESIAN_POINT('',(1.,-6.92820323027551,9.));
#8517=CARTESIAN_POINT('Ctrl Pts',(1.,-6.92820323027551,9.));
#8518=CARTESIAN_POINT('Ctrl Pts',(1.,-6.92820323027551,8.87425193147876));
#8519=CARTESIAN_POINT('Ctrl Pts',(0.974833943897391,-6.93198034025289,8.74024144192777));
#8520=CARTESIAN_POINT('Ctrl Pts',(0.872727208600932,-6.94557411965751,8.49391406486289));
#8521=CARTESIAN_POINT('Ctrl Pts',(0.795795807000654,-6.95518913236708,8.38158224462756));
#8522=CARTESIAN_POINT('Ctrl Pts',(0.618419025069236,-6.97319901589886,8.20420546269614));
#8523=CARTESIAN_POINT('Ctrl Pts',(0.506086655807109,-6.98277103675548,8.12727306529771));
#8524=CARTESIAN_POINT('Ctrl Pts',(0.259757407800085,-6.99626622874452,8.02516560412687));
#8525=CARTESIAN_POINT('Ctrl Pts',(0.125746268276869,-7.,8.));
#8526=CARTESIAN_POINT('Ctrl Pts',(-0.125746268276869,-7.,8.));
#8527=CARTESIAN_POINT('Ctrl Pts',(-0.259757407800085,-6.99626622874452,
8.02516560412687));
#8528=CARTESIAN_POINT('Ctrl Pts',(-0.506086655807109,-6.98277103675548,
8.12727306529771));
#8529=CARTESIAN_POINT('Ctrl Pts',(-0.618419025069236,-6.97319901589886,
8.20420546269614));
#8530=CARTESIAN_POINT('Ctrl Pts',(-0.795795807000653,-6.95518913236708,
8.38158224462756));
#8531=CARTESIAN_POINT('Ctrl Pts',(-0.872727208600933,-6.94557411965751,
8.49391406486289));
#8532=CARTESIAN_POINT('Ctrl Pts',(-0.974833943897392,-6.93198034025289,
8.74024144192777));
#8533=CARTESIAN_POINT('Ctrl Pts',(-1.,-6.92820323027551,8.87425193147876));
#8534=CARTESIAN_POINT('Ctrl Pts',(-1.,-6.92820323027551,9.));
#8535=CARTESIAN_POINT('Ctrl Pts',(-1.,-6.92820323027551,9.));
#8536=CARTESIAN_POINT('Ctrl Pts',(-1.,-6.92820323027551,9.12574806852124));
#8537=CARTESIAN_POINT('Ctrl Pts',(-0.974833943897391,-6.93198034025289,
9.25975855807223));
#8538=CARTESIAN_POINT('Ctrl Pts',(-0.872727208600932,-6.94557411965751,
9.50608593513711));
#8539=CARTESIAN_POINT('Ctrl Pts',(-0.795795807000653,-6.95518913236708,
9.61841775537244));
#8540=CARTESIAN_POINT('Ctrl Pts',(-0.618419025069235,-6.97319901589886,
9.79579453730386));
#8541=CARTESIAN_POINT('Ctrl Pts',(-0.506086655807108,-6.98277103675548,
9.87272693470229));
#8542=CARTESIAN_POINT('Ctrl Pts',(-0.259757407800085,-6.99626622874452,
9.97483439587313));
#8543=CARTESIAN_POINT('Ctrl Pts',(-0.125746268276869,-7.,10.));
#8544=CARTESIAN_POINT('Ctrl Pts',(0.125746268276869,-7.,10.));
#8545=CARTESIAN_POINT('Ctrl Pts',(0.259757407800085,-6.99626622874452,9.97483439587313));
#8546=CARTESIAN_POINT('Ctrl Pts',(0.506086655807109,-6.98277103675548,9.87272693470229));
#8547=CARTESIAN_POINT('Ctrl Pts',(0.618419025069235,-6.97319901589886,9.79579453730386));
#8548=CARTESIAN_POINT('Ctrl Pts',(0.795795807000653,-6.95518913236708,9.61841775537244));
#8549=CARTESIAN_POINT('Ctrl Pts',(0.872727208600933,-6.94557411965751,9.50608593513711));
#8550=CARTESIAN_POINT('Ctrl Pts',(0.974833943897392,-6.93198034025289,9.25975855807223));
#8551=CARTESIAN_POINT('Ctrl Pts',(1.,-6.92820323027551,9.12574806852124));
#8552=CARTESIAN_POINT('Ctrl Pts',(1.,-6.92820323027551,9.));
#8553=CARTESIAN_POINT('Origin',(0.,-6.,10.5));
#8554=CARTESIAN_POINT('',(1.,-6.,6.5));
#8555=CARTESIAN_POINT('',(1.,-6.,14.5));
#8556=CARTESIAN_POINT('',(-1.,-6.,6.5));
#8557=CARTESIAN_POINT('Origin',(0.,-6.,6.5));
#8558=CARTESIAN_POINT('',(-1.,-6.,6.5));
#8559=CARTESIAN_POINT('Origin',(0.,-6.,10.5));
#8560=CARTESIAN_POINT('',(-1.,-6.,12.));
#8561=CARTESIAN_POINT('',(-1.,-6.,6.5));
#8562=CARTESIAN_POINT('',(1.,-6.,12.));
#8563=CARTESIAN_POINT('',(0.,-6.,12.));
#8564=CARTESIAN_POINT('',(1.,-6.,14.5));
#8565=CARTESIAN_POINT('Origin',(0.,0.,6.5));
#8566=CARTESIAN_POINT('',(-1.,-4.89897948556636,6.5));
#8567=CARTESIAN_POINT('',(1.,-4.89897948556636,6.5));
#8568=CARTESIAN_POINT('Ctrl Pts',(-1.,-4.89897948556636,6.5));
#8569=CARTESIAN_POINT('Ctrl Pts',(-1.,-4.89897948556636,6.3740682480366));
#8570=CARTESIAN_POINT('Ctrl Pts',(-0.974762796248615,-4.90433876618447,
6.23998222283811));
#8571=CARTESIAN_POINT('Ctrl Pts',(-0.872605417648384,-4.92354150792771,
5.99370799496995));
#8572=CARTESIAN_POINT('Ctrl Pts',(-0.795703102192089,-4.93709085101933,
5.88148953981899));
#8573=CARTESIAN_POINT('Ctrl Pts',(-0.618515424645094,-4.96240337638318,
5.704301862272));
#8574=CARTESIAN_POINT('Ctrl Pts',(-0.506294861197626,-4.97583347151864,
5.62739565845524));
#8575=CARTESIAN_POINT('Ctrl Pts',(-0.260013306081865,-4.99476188647081,
5.52523545776417));
#8576=CARTESIAN_POINT('Ctrl Pts',(-0.1259246954214,-5.,5.5));
#8577=CARTESIAN_POINT('Ctrl Pts',(0.125924695421399,-5.,5.5));
#8578=CARTESIAN_POINT('Ctrl Pts',(0.260013306081865,-4.99476188647081,5.52523545776417));
#8579=CARTESIAN_POINT('Ctrl Pts',(0.506294861197626,-4.97583347151864,5.62739565845524));
#8580=CARTESIAN_POINT('Ctrl Pts',(0.618515424645094,-4.96240337638318,5.704301862272));
#8581=CARTESIAN_POINT('Ctrl Pts',(0.795703102192088,-4.93709085101933,5.88148953981899));
#8582=CARTESIAN_POINT('Ctrl Pts',(0.872605417648382,-4.92354150792771,5.99370799496995));
#8583=CARTESIAN_POINT('Ctrl Pts',(0.974762796248614,-4.90433876618447,6.23998222283811));
#8584=CARTESIAN_POINT('Ctrl Pts',(1.,-4.89897948556636,6.3740682480366));
#8585=CARTESIAN_POINT('Ctrl Pts',(1.,-4.89897948556636,6.5));
#8586=CARTESIAN_POINT('',(-1.,0.,6.5));
#8587=CARTESIAN_POINT('',(1.,0.,6.5));
#8588=CARTESIAN_POINT('Origin',(1.,0.,6.5));
#8589=CARTESIAN_POINT('',(1.,-4.89897948556636,12.));
#8590=CARTESIAN_POINT('',(1.,-4.89897948556636,5.));
#8591=CARTESIAN_POINT('',(1.,0.,12.));
#8592=CARTESIAN_POINT('Origin',(-1.,0.,14.5));
#8593=CARTESIAN_POINT('',(-1.,-4.89897948556636,12.));
#8594=CARTESIAN_POINT('',(-1.,-4.89897948556636,5.));
#8595=CARTESIAN_POINT('',(-1.,0.,12.));
#8596=CARTESIAN_POINT('Origin',(0.,0.,5.));
#8597=CARTESIAN_POINT('',(-5.,-6.12323399573677E-16,5.));
#8598=CARTESIAN_POINT('Origin',(0.,0.,5.));
#8599=CARTESIAN_POINT('',(-5.,-6.12323399573677E-16,12.));
#8600=CARTESIAN_POINT('',(-5.,-6.12323399573677E-16,5.));
#8601=CARTESIAN_POINT('Origin',(0.,0.,12.));
#8602=CARTESIAN_POINT('Origin',(0.,0.,12.));
#8603=CARTESIAN_POINT('Origin',(0.,0.,5.));
#8604=CARTESIAN_POINT('',(11.9792754136349,-0.704954299427529,5.));
#8605=CARTESIAN_POINT('',(11.9792754136349,-0.704954299427527,0.2));
#8606=CARTESIAN_POINT('',(11.9792754136349,-0.704954299427529,5.));
#8607=CARTESIAN_POINT('',(5.37912937500617,10.726833976852,5.));
#8608=CARTESIAN_POINT('Origin',(0.,0.,5.));
#8609=CARTESIAN_POINT('',(5.37912937500618,10.726833976852,0.2));
#8610=CARTESIAN_POINT('',(5.37912937500617,10.726833976852,5.));
#8611=CARTESIAN_POINT('Origin',(0.,0.,0.2));
#8612=CARTESIAN_POINT('Origin',(0.,0.,5.));
#8613=CARTESIAN_POINT('',(-11.9792754136349,-0.704954299427521,5.));
#8614=CARTESIAN_POINT('',(-11.9792754136349,-0.704954299427494,0.2));
#8615=CARTESIAN_POINT('',(-11.9792754136349,-0.704954299427521,5.));
#8616=CARTESIAN_POINT('',(-5.37912937500617,10.726833976852,0.2));
#8617=CARTESIAN_POINT('Origin',(0.,0.,0.2));
#8618=CARTESIAN_POINT('',(-5.37912937500617,10.726833976852,5.));
#8619=CARTESIAN_POINT('',(-5.37912937500617,10.726833976852,5.));
#8620=CARTESIAN_POINT('Origin',(0.,0.,5.));
#8621=CARTESIAN_POINT('Origin',(0.,0.,5.));
#8622=CARTESIAN_POINT('',(6.60014603862876,-10.0218796774244,5.));
#8623=CARTESIAN_POINT('',(6.60014603862877,-10.0218796774244,0.2));
#8624=CARTESIAN_POINT('',(6.60014603862876,-10.0218796774244,5.));
#8625=CARTESIAN_POINT('',(-6.60014603862878,-10.0218796774244,0.2));
#8626=CARTESIAN_POINT('Origin',(0.,0.,0.2));
#8627=CARTESIAN_POINT('',(-6.60014603862878,-10.0218796774244,5.));
#8628=CARTESIAN_POINT('',(-6.60014603862878,-10.0218796774244,5.));
#8629=CARTESIAN_POINT('Origin',(0.,0.,5.));
#8630=CARTESIAN_POINT('Origin',(0.,0.,0.2));
#8631=CARTESIAN_POINT('',(-13.5,-1.66533453693773E-15,0.2));
#8632=CARTESIAN_POINT('Origin',(0.,0.,0.2));
#8633=CARTESIAN_POINT('Origin',(0.,0.,0.2));
#8634=CARTESIAN_POINT('Origin',(0.,0.,0.2));
#8635=CARTESIAN_POINT('Origin',(0.,0.,0.2));
#8636=CARTESIAN_POINT('Origin',(0.,0.,5.));
#8637=CARTESIAN_POINT('',(-11.9792754136349,-0.70495429942752,-1.5));
#8638=CARTESIAN_POINT('',(-11.9792754136349,-0.704954299427521,5.));
#8639=CARTESIAN_POINT('',(-6.60014603862878,-10.0218796774244,-1.5));
#8640=CARTESIAN_POINT('Origin',(0.,0.,-1.5));
#8641=CARTESIAN_POINT('',(-6.60014603862878,-10.0218796774244,5.));
#8642=CARTESIAN_POINT('Origin',(0.,0.,5.));
#8643=CARTESIAN_POINT('',(5.37912937500617,10.726833976852,-1.5));
#8644=CARTESIAN_POINT('',(5.37912937500617,10.726833976852,5.));
#8645=CARTESIAN_POINT('',(-5.37912937500617,10.726833976852,-1.5));
#8646=CARTESIAN_POINT('Origin',(0.,0.,-1.5));
#8647=CARTESIAN_POINT('',(-5.37912937500617,10.726833976852,5.));
#8648=CARTESIAN_POINT('Origin',(0.,0.,5.));
#8649=CARTESIAN_POINT('',(-6.06863042059311,-5.89037560471066,5.));
#8650=CARTESIAN_POINT('Ctrl Pts',(-6.06863042059311,-5.89037560471066,5.));
#8651=CARTESIAN_POINT('Ctrl Pts',(-6.18294115692138,-6.00132867417749,5.));
#8652=CARTESIAN_POINT('Ctrl Pts',(-6.25574916854265,-6.14973629251005,5.));
#8653=CARTESIAN_POINT('Ctrl Pts',(-6.34958522348951,-6.33256064405531,5.));
#8654=CARTESIAN_POINT('Ctrl Pts',(-6.42989690394213,-6.49149718347625,5.));
#8655=CARTESIAN_POINT('Ctrl Pts',(-6.57404148726985,-6.92443841216413,5.));
#8656=CARTESIAN_POINT('Ctrl Pts',(-6.67668490053576,-7.26884512749233,5.));
#8657=CARTESIAN_POINT('Ctrl Pts',(-6.80496270259299,-8.4372608114701,5.));
#8658=CARTESIAN_POINT('Ctrl Pts',(-6.77273909127515,-9.1969740069116,5.));
#8659=CARTESIAN_POINT('Ctrl Pts',(-6.60014603862878,-10.0218796774244,5.));
#8660=CARTESIAN_POINT('',(-4.62971553586298,-4.49372618847532,5.));
#8661=CARTESIAN_POINT('',(-4.62971553586298,-4.49372618847532,5.));
#8662=CARTESIAN_POINT('',(-4.51042861629926,-3.19779215979849,5.));
#8663=CARTESIAN_POINT('Origin',(-5.32620517920381,-3.77615934370128,5.));
#8664=CARTESIAN_POINT('',(-5.02458355455784,-2.3072496837722,5.));
#8665=CARTESIAN_POINT('Origin',(0.,0.,5.));
#8666=CARTESIAN_POINT('',(-6.20653880480254,-1.76258817211517,5.));
#8667=CARTESIAN_POINT('Origin',(-5.93335250998519,-2.72454931910811,5.));
#8668=CARTESIAN_POINT('',(-8.13553012180811,-2.31040030805734,5.));
#8669=CARTESIAN_POINT('',(-8.13553012180811,-2.31040030805734,5.));
#8670=CARTESIAN_POINT('Ctrl Pts',(-11.9792754136349,-0.704954299427526,
5.));
#8671=CARTESIAN_POINT('Ctrl Pts',(-11.5957187865582,-1.04810301200968,5.));
#8672=CARTESIAN_POINT('Ctrl Pts',(-11.1804727745354,-1.35730649168446,5.));
#8673=CARTESIAN_POINT('Ctrl Pts',(-10.1618489906271,-1.95221245619236,5.));
#8674=CARTESIAN_POINT('Ctrl Pts',(-9.70098587325195,-2.10951926095094,5.));
#8675=CARTESIAN_POINT('Ctrl Pts',(-8.94253026840227,-2.32740085079442,5.));
#8676=CARTESIAN_POINT('Ctrl Pts',(-8.60665429330284,-2.34186126624272,5.));
#8677=CARTESIAN_POINT('Ctrl Pts',(-8.28801320409324,-2.3379034137458,5.));
#8678=CARTESIAN_POINT('Ctrl Pts',(-8.21242123795409,-2.33223653209814,5.));
#8679=CARTESIAN_POINT('Ctrl Pts',(-8.13553012180811,-2.31040030805734,5.));
#8680=CARTESIAN_POINT('',(-2.066899701215,8.20077591276801,5.));
#8681=CARTESIAN_POINT('Ctrl Pts',(-2.066899701215,8.20077591276801,5.));
#8682=CARTESIAN_POINT('Ctrl Pts',(-2.10583250983699,8.35524844908701,5.));
#8683=CARTESIAN_POINT('Ctrl Pts',(-2.19795327161749,8.49250584591636,5.));
#8684=CARTESIAN_POINT('Ctrl Pts',(-2.30936577700739,8.66518242905562,5.));
#8685=CARTESIAN_POINT('Ctrl Pts',(-2.40685301751263,8.81420265426477,5.));
#8686=CARTESIAN_POINT('Ctrl Pts',(-2.70971882823706,9.1555061395873,5.));
#8687=CARTESIAN_POINT('Ctrl Pts',(-2.9566620863145,9.4166013006736,5.));
#8688=CARTESIAN_POINT('Ctrl Pts',(-3.90440084957731,10.111900977829,5.));
#8689=CARTESIAN_POINT('Ctrl Pts',(-4.57844358199661,10.4638511096066,5.));
#8690=CARTESIAN_POINT('Ctrl Pts',(-5.37912937500617,10.726833976852,5.));
#8691=CARTESIAN_POINT('',(-1.57682326893955,6.25631436059049,5.));
#8692=CARTESIAN_POINT('',(-1.57682326893955,6.25631436059049,5.));
#8693=CARTESIAN_POINT('',(-0.514154938258575,5.5050418435707,5.));
#8694=CARTESIAN_POINT('Origin',(-0.607147330781379,6.50070866280939,5.));
#8695=CARTESIAN_POINT('',(0.514154938258576,5.5050418435707,5.));
#8696=CARTESIAN_POINT('Origin',(0.,0.,5.));
#8697=CARTESIAN_POINT('',(1.57682326893955,6.25631436059049,5.));
#8698=CARTESIAN_POINT('Origin',(0.60714733078138,6.50070866280939,5.));
#8699=CARTESIAN_POINT('',(2.066899701215,8.20077591276801,5.));
#8700=CARTESIAN_POINT('',(2.066899701215,8.20077591276801,5.));
#8701=CARTESIAN_POINT('Ctrl Pts',(5.37912937500617,10.726833976852,5.));
#8702=CARTESIAN_POINT('Ctrl Pts',(4.89017555917646,10.5662385503313,5.));
#8703=CARTESIAN_POINT('Ctrl Pts',(4.41477448478803,10.3612266949343,5.));
#8704=CARTESIAN_POINT('Ctrl Pts',(3.39025891472665,9.77652560343359,5.));
#8705=CARTESIAN_POINT('Ctrl Pts',(3.02359566700368,9.45605983859608,5.));
#8706=CARTESIAN_POINT('Ctrl Pts',(2.4556768726076,8.90815881192699,5.));
#8707=CARTESIAN_POINT('Ctrl Pts',(2.27521579794331,8.62451189270667,5.));
#8708=CARTESIAN_POINT('Ctrl Pts',(2.11932285414767,8.34658168851712,5.));
#8709=CARTESIAN_POINT('Ctrl Pts',(2.08643453454576,8.27828368469551,5.));
#8710=CARTESIAN_POINT('Ctrl Pts',(2.066899701215,8.20077591276801,5.));
#8711=CARTESIAN_POINT('',(8.13553012180811,-2.31040030805735,5.));
#8712=CARTESIAN_POINT('Ctrl Pts',(8.13553012180811,-2.31040030805735,5.));
#8713=CARTESIAN_POINT('Ctrl Pts',(8.28877366675838,-2.35391977490952,5.));
#8714=CARTESIAN_POINT('Ctrl Pts',(8.45370244016016,-2.34276955340631,5.));
#8715=CARTESIAN_POINT('Ctrl Pts',(8.65895100049858,-2.33262178500872,5.));
#8716=CARTESIAN_POINT('Ctrl Pts',(8.83674992145612,-2.32270547079077,5.));
#8717=CARTESIAN_POINT('Ctrl Pts',(9.28376031551307,-2.23106772742579,5.));
#8718=CARTESIAN_POINT('Ctrl Pts',(9.63334698685416,-2.14775617318037,5.));
#8719=CARTESIAN_POINT('Ctrl Pts',(10.70936355228,-1.67464016656206,5.));
#8720=CARTESIAN_POINT('Ctrl Pts',(11.3511826734672,-1.26687710288273,5.));
#8721=CARTESIAN_POINT('Ctrl Pts',(11.9792754136349,-0.704954299427529,5.));
#8722=CARTESIAN_POINT('',(6.20653880480254,-1.76258817211517,5.));
#8723=CARTESIAN_POINT('',(6.20653880480254,-1.76258817211517,5.));
#8724=CARTESIAN_POINT('',(5.02458355455784,-2.3072496837722,5.));
#8725=CARTESIAN_POINT('Origin',(5.93335250998519,-2.72454931910811,5.));
#8726=CARTESIAN_POINT('',(4.51042861629926,-3.1977921597985,5.));
#8727=CARTESIAN_POINT('Origin',(0.,0.,5.));
#8728=CARTESIAN_POINT('',(4.62971553586298,-4.49372618847532,5.));
#8729=CARTESIAN_POINT('Origin',(5.32620517920381,-3.77615934370129,5.));
#8730=CARTESIAN_POINT('',(6.06863042059311,-5.89037560471067,5.));
#8731=CARTESIAN_POINT('',(6.06863042059311,-5.89037560471067,5.));
#8732=CARTESIAN_POINT('Ctrl Pts',(6.60014603862877,-10.0218796774244,5.));
#8733=CARTESIAN_POINT('Ctrl Pts',(6.70554322747048,-9.51813553825663,5.));
#8734=CARTESIAN_POINT('Ctrl Pts',(6.76569828978878,-9.00392020319332,5.));
#8735=CARTESIAN_POINT('Ctrl Pts',(6.77159007595975,-7.82431314719937,5.));
#8736=CARTESIAN_POINT('Ctrl Pts',(6.67739020636713,-7.34654057745018,5.));
#8737=CARTESIAN_POINT('Ctrl Pts',(6.48685339577297,-6.58075796113559,5.));
#8738=CARTESIAN_POINT('Ctrl Pts',(6.33143849535284,-6.28265062646335,5.));
#8739=CARTESIAN_POINT('Ctrl Pts',(6.16869034994494,-6.00867827477288,5.));
#8740=CARTESIAN_POINT('Ctrl Pts',(6.12598670340806,-5.94604715259793,5.));
#8741=CARTESIAN_POINT('Ctrl Pts',(6.06863042059311,-5.89037560471067,5.));
#8742=CARTESIAN_POINT('Origin',(0.,0.,6.));
#8743=CARTESIAN_POINT('',(7.,-8.57252759403147E-16,12.));
#8744=CARTESIAN_POINT('Origin',(0.,0.,12.));
#8745=CARTESIAN_POINT('',(7.,-8.57252759403147E-16,6.));
#8746=CARTESIAN_POINT('',(7.,8.57252759403147E-16,6.));
#8747=CARTESIAN_POINT('Origin',(0.,0.,6.));
#8748=CARTESIAN_POINT('Origin',(0.,0.,12.));
#8749=CARTESIAN_POINT('Origin',(0.,0.,5.));
#8750=CARTESIAN_POINT('',(-13.5,-1.65327317884893E-15,6.));
#8751=CARTESIAN_POINT('Origin',(0.,0.,6.));
#8752=CARTESIAN_POINT('',(-13.5,-1.65327317884893E-15,5.));
#8753=CARTESIAN_POINT('Origin',(0.,0.,6.));
#8754=CARTESIAN_POINT('Origin',(0.,0.,5.));
#8755=CARTESIAN_POINT('',(-4.51042861629926,-3.19779215979849,-1.5));
#8756=CARTESIAN_POINT('',(-4.51042861629926,-3.19779215979849,5.));
#8757=CARTESIAN_POINT('',(-5.02458355455784,-2.3072496837722,-1.5));
#8758=CARTESIAN_POINT('Origin',(0.,0.,-1.5));
#8759=CARTESIAN_POINT('',(-5.02458355455784,-2.3072496837722,5.));
#8760=CARTESIAN_POINT('Origin',(-5.93335250998519,-2.72454931910811,5.));
#8761=CARTESIAN_POINT('',(-6.20653880480254,-1.76258817211517,-1.5));
#8762=CARTESIAN_POINT('Origin',(-5.93335250998519,-2.72454931910811,-1.5));
#8763=CARTESIAN_POINT('',(-6.20653880480254,-1.76258817211517,5.));
#8764=CARTESIAN_POINT('Origin',(-8.13553012180811,-2.31040030805734,5.));
#8765=CARTESIAN_POINT('',(-8.13553012180811,-2.31040030805734,-1.5));
#8766=CARTESIAN_POINT('',(-8.13553012180811,-2.31040030805734,-1.5));
#8767=CARTESIAN_POINT('',(-8.13553012180811,-2.31040030805734,5.));
#8768=CARTESIAN_POINT('Ctrl Pts',(-11.9792754136349,-0.704954299427526,
5.));
#8769=CARTESIAN_POINT('Ctrl Pts',(-11.9792754136349,-0.704954299427526,
-2.8));
#8770=CARTESIAN_POINT('Ctrl Pts',(-11.5957187865582,-1.04810301200968,5.));
#8771=CARTESIAN_POINT('Ctrl Pts',(-11.5957187865582,-1.04810301200968,-2.8));
#8772=CARTESIAN_POINT('Ctrl Pts',(-11.1804727745354,-1.35730649168446,5.));
#8773=CARTESIAN_POINT('Ctrl Pts',(-11.1804727745354,-1.35730649168446,-2.8));
#8774=CARTESIAN_POINT('Ctrl Pts',(-10.1618489906271,-1.95221245619236,5.));
#8775=CARTESIAN_POINT('Ctrl Pts',(-10.1618489906271,-1.95221245619236,-2.8));
#8776=CARTESIAN_POINT('Ctrl Pts',(-9.70098587325195,-2.10951926095094,5.));
#8777=CARTESIAN_POINT('Ctrl Pts',(-9.70098587325195,-2.10951926095094,-2.8));
#8778=CARTESIAN_POINT('Ctrl Pts',(-8.94253026840227,-2.32740085079442,5.));
#8779=CARTESIAN_POINT('Ctrl Pts',(-8.94253026840227,-2.32740085079442,-2.8));
#8780=CARTESIAN_POINT('Ctrl Pts',(-8.60665429330284,-2.34186126624272,5.));
#8781=CARTESIAN_POINT('Ctrl Pts',(-8.60665429330284,-2.34186126624272,-2.8));
#8782=CARTESIAN_POINT('Ctrl Pts',(-8.28801320409324,-2.3379034137458,5.));
#8783=CARTESIAN_POINT('Ctrl Pts',(-8.28801320409324,-2.3379034137458,-2.8));
#8784=CARTESIAN_POINT('Ctrl Pts',(-8.21242123795409,-2.33223653209814,5.));
#8785=CARTESIAN_POINT('Ctrl Pts',(-8.21242123795409,-2.33223653209814,-2.8));
#8786=CARTESIAN_POINT('Ctrl Pts',(-8.13553012180811,-2.31040030805734,5.));
#8787=CARTESIAN_POINT('Ctrl Pts',(-8.13553012180811,-2.31040030805734,-2.8));
#8788=CARTESIAN_POINT('Ctrl Pts',(-11.9792754136349,-0.704954299427526,
-1.5));
#8789=CARTESIAN_POINT('Ctrl Pts',(-11.5957187865582,-1.04810301200968,-1.5));
#8790=CARTESIAN_POINT('Ctrl Pts',(-11.1804727745354,-1.35730649168446,-1.5));
#8791=CARTESIAN_POINT('Ctrl Pts',(-10.1618489906271,-1.95221245619236,-1.5));
#8792=CARTESIAN_POINT('Ctrl Pts',(-9.70098587325195,-2.10951926095094,-1.5));
#8793=CARTESIAN_POINT('Ctrl Pts',(-8.94253026840227,-2.32740085079442,-1.5));
#8794=CARTESIAN_POINT('Ctrl Pts',(-8.60665429330284,-2.34186126624272,-1.5));
#8795=CARTESIAN_POINT('Ctrl Pts',(-8.28801320409324,-2.3379034137458,-1.5));
#8796=CARTESIAN_POINT('Ctrl Pts',(-8.21242123795409,-2.33223653209814,-1.5));
#8797=CARTESIAN_POINT('Ctrl Pts',(-8.13553012180811,-2.31040030805734,-1.5));
#8798=CARTESIAN_POINT('Ctrl Pts',(-6.06863042059311,-5.89037560471066,5.));
#8799=CARTESIAN_POINT('Ctrl Pts',(-6.06863042059311,-5.89037560471066,-2.8));
#8800=CARTESIAN_POINT('Ctrl Pts',(-6.18294115692138,-6.00132867417749,5.));
#8801=CARTESIAN_POINT('Ctrl Pts',(-6.18294115692138,-6.00132867417749,-2.8));
#8802=CARTESIAN_POINT('Ctrl Pts',(-6.25574916854265,-6.14973629251005,5.));
#8803=CARTESIAN_POINT('Ctrl Pts',(-6.25574916854265,-6.14973629251005,-2.8));
#8804=CARTESIAN_POINT('Ctrl Pts',(-6.34958522348951,-6.33256064405531,5.));
#8805=CARTESIAN_POINT('Ctrl Pts',(-6.34958522348951,-6.33256064405531,-2.8));
#8806=CARTESIAN_POINT('Ctrl Pts',(-6.42989690394213,-6.49149718347625,5.));
#8807=CARTESIAN_POINT('Ctrl Pts',(-6.42989690394213,-6.49149718347625,-2.8));
#8808=CARTESIAN_POINT('Ctrl Pts',(-6.57404148726985,-6.92443841216413,5.));
#8809=CARTESIAN_POINT('Ctrl Pts',(-6.57404148726985,-6.92443841216413,-2.8));
#8810=CARTESIAN_POINT('Ctrl Pts',(-6.67668490053576,-7.26884512749233,5.));
#8811=CARTESIAN_POINT('Ctrl Pts',(-6.67668490053576,-7.26884512749233,-2.8));
#8812=CARTESIAN_POINT('Ctrl Pts',(-6.80496270259299,-8.4372608114701,5.));
#8813=CARTESIAN_POINT('Ctrl Pts',(-6.80496270259299,-8.4372608114701,-2.8));
#8814=CARTESIAN_POINT('Ctrl Pts',(-6.77273909127515,-9.1969740069116,5.));
#8815=CARTESIAN_POINT('Ctrl Pts',(-6.77273909127515,-9.1969740069116,-2.8));
#8816=CARTESIAN_POINT('Ctrl Pts',(-6.60014603862878,-10.0218796774244,5.));
#8817=CARTESIAN_POINT('Ctrl Pts',(-6.60014603862878,-10.0218796774244,-2.8));
#8818=CARTESIAN_POINT('',(-6.06863042059311,-5.89037560471066,-1.5));
#8819=CARTESIAN_POINT('Ctrl Pts',(-6.06863042059311,-5.89037560471066,-1.5));
#8820=CARTESIAN_POINT('Ctrl Pts',(-6.18294115692138,-6.00132867417749,-1.5));
#8821=CARTESIAN_POINT('Ctrl Pts',(-6.25574916854265,-6.14973629251005,-1.5));
#8822=CARTESIAN_POINT('Ctrl Pts',(-6.34958522348951,-6.33256064405531,-1.5));
#8823=CARTESIAN_POINT('Ctrl Pts',(-6.42989690394213,-6.49149718347625,-1.5));
#8824=CARTESIAN_POINT('Ctrl Pts',(-6.57404148726985,-6.92443841216413,-1.5));
#8825=CARTESIAN_POINT('Ctrl Pts',(-6.67668490053576,-7.26884512749233,-1.5));
#8826=CARTESIAN_POINT('Ctrl Pts',(-6.80496270259299,-8.4372608114701,-1.5));
#8827=CARTESIAN_POINT('Ctrl Pts',(-6.77273909127515,-9.1969740069116,-1.5));
#8828=CARTESIAN_POINT('Ctrl Pts',(-6.60014603862878,-10.0218796774244,-1.5));
#8829=CARTESIAN_POINT('',(-6.06863042059311,-5.89037560471066,5.));
#8830=CARTESIAN_POINT('Origin',(-4.62971553586298,-4.49372618847532,5.));
#8831=CARTESIAN_POINT('',(-4.62971553586298,-4.49372618847532,-1.5));
#8832=CARTESIAN_POINT('',(-4.62971553586298,-4.49372618847532,-1.5));
#8833=CARTESIAN_POINT('',(-4.62971553586298,-4.49372618847532,5.));
#8834=CARTESIAN_POINT('Origin',(-5.32620517920381,-3.77615934370128,5.));
#8835=CARTESIAN_POINT('Origin',(-5.32620517920381,-3.77615934370128,-1.5));
#8836=CARTESIAN_POINT('Origin',(-8.15362319838813,-5.36431270931319,-1.5));
#8837=CARTESIAN_POINT('Origin',(0.,0.,5.));
#8838=CARTESIAN_POINT('',(-0.514154938258575,5.5050418435707,-1.5));
#8839=CARTESIAN_POINT('',(-0.514154938258575,5.5050418435707,5.));
#8840=CARTESIAN_POINT('',(0.514154938258576,5.5050418435707,-1.5));
#8841=CARTESIAN_POINT('Origin',(0.,0.,-1.5));
#8842=CARTESIAN_POINT('',(0.514154938258576,5.5050418435707,5.));
#8843=CARTESIAN_POINT('Origin',(0.60714733078138,6.50070866280939,5.));
#8844=CARTESIAN_POINT('',(1.57682326893956,6.25631436059049,-1.5));
#8845=CARTESIAN_POINT('Origin',(0.60714733078138,6.50070866280939,-1.5));
#8846=CARTESIAN_POINT('',(1.57682326893955,6.25631436059049,5.));
#8847=CARTESIAN_POINT('Origin',(2.066899701215,8.20077591276801,5.));
#8848=CARTESIAN_POINT('',(2.066899701215,8.20077591276801,-1.5));
#8849=CARTESIAN_POINT('',(2.066899701215,8.20077591276801,-1.5));
#8850=CARTESIAN_POINT('',(2.066899701215,8.20077591276801,5.));
#8851=CARTESIAN_POINT('Ctrl Pts',(5.37912937500617,10.726833976852,5.));
#8852=CARTESIAN_POINT('Ctrl Pts',(5.37912937500617,10.726833976852,-2.8));
#8853=CARTESIAN_POINT('Ctrl Pts',(4.89017555917646,10.5662385503313,5.));
#8854=CARTESIAN_POINT('Ctrl Pts',(4.89017555917646,10.5662385503313,-2.8));
#8855=CARTESIAN_POINT('Ctrl Pts',(4.41477448478803,10.3612266949343,5.));
#8856=CARTESIAN_POINT('Ctrl Pts',(4.41477448478803,10.3612266949343,-2.8));
#8857=CARTESIAN_POINT('Ctrl Pts',(3.39025891472665,9.77652560343359,5.));
#8858=CARTESIAN_POINT('Ctrl Pts',(3.39025891472665,9.77652560343359,-2.8));
#8859=CARTESIAN_POINT('Ctrl Pts',(3.02359566700368,9.45605983859608,5.));
#8860=CARTESIAN_POINT('Ctrl Pts',(3.02359566700368,9.45605983859608,-2.8));
#8861=CARTESIAN_POINT('Ctrl Pts',(2.4556768726076,8.90815881192699,5.));
#8862=CARTESIAN_POINT('Ctrl Pts',(2.4556768726076,8.90815881192699,-2.8));
#8863=CARTESIAN_POINT('Ctrl Pts',(2.27521579794331,8.62451189270667,5.));
#8864=CARTESIAN_POINT('Ctrl Pts',(2.27521579794331,8.62451189270667,-2.8));
#8865=CARTESIAN_POINT('Ctrl Pts',(2.11932285414767,8.34658168851712,5.));
#8866=CARTESIAN_POINT('Ctrl Pts',(2.11932285414767,8.34658168851712,-2.8));
#8867=CARTESIAN_POINT('Ctrl Pts',(2.08643453454576,8.27828368469551,5.));
#8868=CARTESIAN_POINT('Ctrl Pts',(2.08643453454576,8.27828368469551,-2.8));
#8869=CARTESIAN_POINT('Ctrl Pts',(2.066899701215,8.20077591276801,5.));
#8870=CARTESIAN_POINT('Ctrl Pts',(2.066899701215,8.20077591276801,-2.8));
#8871=CARTESIAN_POINT('Ctrl Pts',(5.37912937500617,10.726833976852,-1.5));
#8872=CARTESIAN_POINT('Ctrl Pts',(4.89017555917646,10.5662385503313,-1.5));
#8873=CARTESIAN_POINT('Ctrl Pts',(4.41477448478803,10.3612266949343,-1.5));
#8874=CARTESIAN_POINT('Ctrl Pts',(3.39025891472665,9.77652560343359,-1.5));
#8875=CARTESIAN_POINT('Ctrl Pts',(3.02359566700368,9.45605983859608,-1.5));
#8876=CARTESIAN_POINT('Ctrl Pts',(2.4556768726076,8.90815881192699,-1.5));
#8877=CARTESIAN_POINT('Ctrl Pts',(2.27521579794331,8.62451189270667,-1.5));
#8878=CARTESIAN_POINT('Ctrl Pts',(2.11932285414767,8.34658168851712,-1.5));
#8879=CARTESIAN_POINT('Ctrl Pts',(2.08643453454576,8.27828368469551,-1.5));
#8880=CARTESIAN_POINT('Ctrl Pts',(2.066899701215,8.20077591276801,-1.5));
#8881=CARTESIAN_POINT('Ctrl Pts',(-2.066899701215,8.20077591276801,5.));
#8882=CARTESIAN_POINT('Ctrl Pts',(-2.066899701215,8.20077591276801,-2.8));
#8883=CARTESIAN_POINT('Ctrl Pts',(-2.10583250983699,8.35524844908701,5.));
#8884=CARTESIAN_POINT('Ctrl Pts',(-2.10583250983699,8.35524844908701,-2.8));
#8885=CARTESIAN_POINT('Ctrl Pts',(-2.19795327161749,8.49250584591636,5.));
#8886=CARTESIAN_POINT('Ctrl Pts',(-2.19795327161749,8.49250584591636,-2.8));
#8887=CARTESIAN_POINT('Ctrl Pts',(-2.30936577700739,8.66518242905562,5.));
#8888=CARTESIAN_POINT('Ctrl Pts',(-2.30936577700739,8.66518242905562,-2.8));
#8889=CARTESIAN_POINT('Ctrl Pts',(-2.40685301751263,8.81420265426477,5.));
#8890=CARTESIAN_POINT('Ctrl Pts',(-2.40685301751263,8.81420265426477,-2.8));
#8891=CARTESIAN_POINT('Ctrl Pts',(-2.70971882823706,9.1555061395873,5.));
#8892=CARTESIAN_POINT('Ctrl Pts',(-2.70971882823706,9.1555061395873,-2.8));
#8893=CARTESIAN_POINT('Ctrl Pts',(-2.9566620863145,9.4166013006736,5.));
#8894=CARTESIAN_POINT('Ctrl Pts',(-2.9566620863145,9.4166013006736,-2.8));
#8895=CARTESIAN_POINT('Ctrl Pts',(-3.90440084957731,10.111900977829,5.));
#8896=CARTESIAN_POINT('Ctrl Pts',(-3.90440084957731,10.111900977829,-2.8));
#8897=CARTESIAN_POINT('Ctrl Pts',(-4.57844358199661,10.4638511096066,5.));
#8898=CARTESIAN_POINT('Ctrl Pts',(-4.57844358199661,10.4638511096066,-2.8));
#8899=CARTESIAN_POINT('Ctrl Pts',(-5.37912937500617,10.726833976852,5.));
#8900=CARTESIAN_POINT('Ctrl Pts',(-5.37912937500617,10.726833976852,-2.8));
#8901=CARTESIAN_POINT('',(-2.066899701215,8.20077591276801,-1.5));
#8902=CARTESIAN_POINT('Ctrl Pts',(-2.066899701215,8.20077591276801,-1.5));
#8903=CARTESIAN_POINT('Ctrl Pts',(-2.10583250983699,8.35524844908701,-1.5));
#8904=CARTESIAN_POINT('Ctrl Pts',(-2.19795327161749,8.49250584591636,-1.5));
#8905=CARTESIAN_POINT('Ctrl Pts',(-2.30936577700739,8.66518242905562,-1.5));
#8906=CARTESIAN_POINT('Ctrl Pts',(-2.40685301751263,8.81420265426477,-1.5));
#8907=CARTESIAN_POINT('Ctrl Pts',(-2.70971882823706,9.1555061395873,-1.5));
#8908=CARTESIAN_POINT('Ctrl Pts',(-2.9566620863145,9.4166013006736,-1.5));
#8909=CARTESIAN_POINT('Ctrl Pts',(-3.90440084957731,10.111900977829,-1.5));
#8910=CARTESIAN_POINT('Ctrl Pts',(-4.57844358199661,10.4638511096066,-1.5));
#8911=CARTESIAN_POINT('Ctrl Pts',(-5.37912937500617,10.726833976852,-1.5));
#8912=CARTESIAN_POINT('',(-2.066899701215,8.20077591276801,5.));
#8913=CARTESIAN_POINT('Origin',(-1.57682326893955,6.25631436059049,5.));
#8914=CARTESIAN_POINT('',(-1.57682326893955,6.25631436059049,-1.5));
#8915=CARTESIAN_POINT('',(-1.57682326893955,6.25631436059049,-1.5));
#8916=CARTESIAN_POINT('',(-1.57682326893955,6.25631436059049,5.));
#8917=CARTESIAN_POINT('Origin',(-0.607147330781379,6.50070866280939,5.));
#8918=CARTESIAN_POINT('Origin',(-0.607147330781379,6.50070866280939,-1.5));
#8919=CARTESIAN_POINT('Origin',(-0.000895720887666984,8.7503543314047,-1.5));
#8920=CARTESIAN_POINT('Origin',(0.,0.,5.));
#8921=CARTESIAN_POINT('',(5.02458355455784,-2.3072496837722,-1.5));
#8922=CARTESIAN_POINT('',(5.02458355455784,-2.3072496837722,5.));
#8923=CARTESIAN_POINT('',(4.51042861629926,-3.1977921597985,-1.5));
#8924=CARTESIAN_POINT('Origin',(0.,0.,-1.5));
#8925=CARTESIAN_POINT('',(4.51042861629926,-3.1977921597985,5.));
#8926=CARTESIAN_POINT('Origin',(5.32620517920381,-3.77615934370129,5.));
#8927=CARTESIAN_POINT('',(4.62971553586298,-4.49372618847532,-1.5));
#8928=CARTESIAN_POINT('Origin',(5.32620517920381,-3.77615934370129,-1.5));
#8929=CARTESIAN_POINT('',(4.62971553586298,-4.49372618847532,5.));
#8930=CARTESIAN_POINT('Origin',(6.06863042059311,-5.89037560471067,5.));
#8931=CARTESIAN_POINT('',(6.06863042059311,-5.89037560471067,-1.5));
#8932=CARTESIAN_POINT('',(6.06863042059311,-5.89037560471067,-1.5));
#8933=CARTESIAN_POINT('',(6.06863042059311,-5.89037560471067,5.));
#8934=CARTESIAN_POINT('Ctrl Pts',(6.60014603862877,-10.0218796774244,5.));
#8935=CARTESIAN_POINT('Ctrl Pts',(6.60014603862877,-10.0218796774244,-2.8));
#8936=CARTESIAN_POINT('Ctrl Pts',(6.70554322747048,-9.51813553825663,5.));
#8937=CARTESIAN_POINT('Ctrl Pts',(6.70554322747048,-9.51813553825663,-2.8));
#8938=CARTESIAN_POINT('Ctrl Pts',(6.76569828978878,-9.00392020319332,5.));
#8939=CARTESIAN_POINT('Ctrl Pts',(6.76569828978878,-9.00392020319332,-2.8));
#8940=CARTESIAN_POINT('Ctrl Pts',(6.77159007595975,-7.82431314719937,5.));
#8941=CARTESIAN_POINT('Ctrl Pts',(6.77159007595975,-7.82431314719937,-2.8));
#8942=CARTESIAN_POINT('Ctrl Pts',(6.67739020636713,-7.34654057745018,5.));
#8943=CARTESIAN_POINT('Ctrl Pts',(6.67739020636713,-7.34654057745018,-2.8));
#8944=CARTESIAN_POINT('Ctrl Pts',(6.48685339577297,-6.58075796113559,5.));
#8945=CARTESIAN_POINT('Ctrl Pts',(6.48685339577297,-6.58075796113559,-2.8));
#8946=CARTESIAN_POINT('Ctrl Pts',(6.33143849535284,-6.28265062646335,5.));
#8947=CARTESIAN_POINT('Ctrl Pts',(6.33143849535284,-6.28265062646335,-2.8));
#8948=CARTESIAN_POINT('Ctrl Pts',(6.16869034994494,-6.00867827477288,5.));
#8949=CARTESIAN_POINT('Ctrl Pts',(6.16869034994494,-6.00867827477288,-2.8));
#8950=CARTESIAN_POINT('Ctrl Pts',(6.12598670340806,-5.94604715259793,5.));
#8951=CARTESIAN_POINT('Ctrl Pts',(6.12598670340806,-5.94604715259793,-2.8));
#8952=CARTESIAN_POINT('Ctrl Pts',(6.06863042059311,-5.89037560471067,5.));
#8953=CARTESIAN_POINT('Ctrl Pts',(6.06863042059311,-5.89037560471067,-2.8));
#8954=CARTESIAN_POINT('',(6.60014603862876,-10.0218796774244,-1.5));
#8955=CARTESIAN_POINT('Ctrl Pts',(6.60014603862877,-10.0218796774244,-1.5));
#8956=CARTESIAN_POINT('Ctrl Pts',(6.70554322747048,-9.51813553825663,-1.5));
#8957=CARTESIAN_POINT('Ctrl Pts',(6.76569828978878,-9.00392020319332,-1.5));
#8958=CARTESIAN_POINT('Ctrl Pts',(6.77159007595975,-7.82431314719937,-1.5));
#8959=CARTESIAN_POINT('Ctrl Pts',(6.67739020636713,-7.34654057745018,-1.5));
#8960=CARTESIAN_POINT('Ctrl Pts',(6.48685339577297,-6.58075796113559,-1.5));
#8961=CARTESIAN_POINT('Ctrl Pts',(6.33143849535284,-6.28265062646335,-1.5));
#8962=CARTESIAN_POINT('Ctrl Pts',(6.16869034994494,-6.00867827477288,-1.5));
#8963=CARTESIAN_POINT('Ctrl Pts',(6.12598670340806,-5.94604715259793,-1.5));
#8964=CARTESIAN_POINT('Ctrl Pts',(6.06863042059311,-5.89037560471067,-1.5));
#8965=CARTESIAN_POINT('',(6.60014603862876,-10.0218796774244,5.));
#8966=CARTESIAN_POINT('Origin',(0.,0.,5.));
#8967=CARTESIAN_POINT('',(11.9792754136349,-0.704954299427529,-1.5));
#8968=CARTESIAN_POINT('Origin',(0.,0.,-1.5));
#8969=CARTESIAN_POINT('',(11.9792754136349,-0.704954299427529,5.));
#8970=CARTESIAN_POINT('Ctrl Pts',(8.13553012180811,-2.31040030805735,5.));
#8971=CARTESIAN_POINT('Ctrl Pts',(8.13553012180811,-2.31040030805735,-2.8));
#8972=CARTESIAN_POINT('Ctrl Pts',(8.28877366675838,-2.35391977490952,5.));
#8973=CARTESIAN_POINT('Ctrl Pts',(8.28877366675838,-2.35391977490952,-2.8));
#8974=CARTESIAN_POINT('Ctrl Pts',(8.45370244016016,-2.34276955340631,5.));
#8975=CARTESIAN_POINT('Ctrl Pts',(8.45370244016016,-2.34276955340631,-2.8));
#8976=CARTESIAN_POINT('Ctrl Pts',(8.65895100049858,-2.33262178500872,5.));
#8977=CARTESIAN_POINT('Ctrl Pts',(8.65895100049858,-2.33262178500872,-2.8));
#8978=CARTESIAN_POINT('Ctrl Pts',(8.83674992145612,-2.32270547079077,5.));
#8979=CARTESIAN_POINT('Ctrl Pts',(8.83674992145612,-2.32270547079077,-2.8));
#8980=CARTESIAN_POINT('Ctrl Pts',(9.28376031551307,-2.23106772742579,5.));
#8981=CARTESIAN_POINT('Ctrl Pts',(9.28376031551307,-2.23106772742579,-2.8));
#8982=CARTESIAN_POINT('Ctrl Pts',(9.63334698685416,-2.14775617318037,5.));
#8983=CARTESIAN_POINT('Ctrl Pts',(9.63334698685416,-2.14775617318037,-2.8));
#8984=CARTESIAN_POINT('Ctrl Pts',(10.70936355228,-1.67464016656206,5.));
#8985=CARTESIAN_POINT('Ctrl Pts',(10.70936355228,-1.67464016656206,-2.8));
#8986=CARTESIAN_POINT('Ctrl Pts',(11.3511826734672,-1.26687710288273,5.));
#8987=CARTESIAN_POINT('Ctrl Pts',(11.3511826734672,-1.26687710288273,-2.8));
#8988=CARTESIAN_POINT('Ctrl Pts',(11.9792754136349,-0.704954299427529,5.));
#8989=CARTESIAN_POINT('Ctrl Pts',(11.9792754136349,-0.704954299427529,-2.8));
#8990=CARTESIAN_POINT('',(8.13553012180811,-2.31040030805735,-1.5));
#8991=CARTESIAN_POINT('Ctrl Pts',(8.13553012180811,-2.31040030805735,-1.5));
#8992=CARTESIAN_POINT('Ctrl Pts',(8.28877366675838,-2.35391977490952,-1.5));
#8993=CARTESIAN_POINT('Ctrl Pts',(8.45370244016016,-2.34276955340631,-1.5));
#8994=CARTESIAN_POINT('Ctrl Pts',(8.65895100049858,-2.33262178500872,-1.5));
#8995=CARTESIAN_POINT('Ctrl Pts',(8.83674992145612,-2.32270547079077,-1.5));
#8996=CARTESIAN_POINT('Ctrl Pts',(9.28376031551307,-2.23106772742579,-1.5));
#8997=CARTESIAN_POINT('Ctrl Pts',(9.63334698685416,-2.14775617318037,-1.5));
#8998=CARTESIAN_POINT('Ctrl Pts',(10.70936355228,-1.67464016656206,-1.5));
#8999=CARTESIAN_POINT('Ctrl Pts',(11.3511826734672,-1.26687710288273,-1.5));
#9000=CARTESIAN_POINT('Ctrl Pts',(11.9792754136349,-0.704954299427529,-1.5));
#9001=CARTESIAN_POINT('',(8.13553012180811,-2.31040030805735,5.));
#9002=CARTESIAN_POINT('Origin',(6.20653880480254,-1.76258817211517,5.));
#9003=CARTESIAN_POINT('',(6.20653880480254,-1.76258817211517,-1.5));
#9004=CARTESIAN_POINT('',(6.20653880480254,-1.76258817211517,-1.5));
#9005=CARTESIAN_POINT('',(6.20653880480254,-1.76258817211517,5.));
#9006=CARTESIAN_POINT('Origin',(5.93335250998519,-2.72454931910811,5.));
#9007=CARTESIAN_POINT('Origin',(5.93335250998519,-2.72454931910811,-1.5));
#9008=CARTESIAN_POINT('Origin',(8.15451891927535,-5.36252126753871,-1.5));
#9803=UNCERTAINTY_MEASURE_WITH_UNIT(LENGTH_MEASURE(0.01),#9823,
'DISTANCE_ACCURACY_VALUE',
'Maximum model space distance between geometric entities at asserted c
onnectivities');
#9811=UNCERTAINTY_MEASURE_WITH_UNIT(LENGTH_MEASURE(0.01),#9823,
'DISTANCE_ACCURACY_VALUE',
'Maximum model space distance between geometric entities at asserted c
onnectivities');
#9814=(
GEOMETRIC_REPRESENTATION_CONTEXT(3)
GLOBAL_UNCERTAINTY_ASSIGNED_CONTEXT((#9803))
GLOBAL_UNIT_ASSIGNED_CONTEXT((#9823,#9825,#9826))
REPRESENTATION_CONTEXT('','3D')
);
#9822=(
GEOMETRIC_REPRESENTATION_CONTEXT(3)
GLOBAL_UNCERTAINTY_ASSIGNED_CONTEXT((#9811))
GLOBAL_UNIT_ASSIGNED_CONTEXT((#9823,#9825,#9826))
REPRESENTATION_CONTEXT('','3D')
);
#9823=(
LENGTH_UNIT()
NAMED_UNIT(*)
SI_UNIT(.MILLI.,.METRE.)
);
#9825=(
NAMED_UNIT(*)
PLANE_ANGLE_UNIT()
SI_UNIT($,.RADIAN.)
);
#9826=(
NAMED_UNIT(*)
SI_UNIT($,.STERADIAN.)
SOLID_ANGLE_UNIT()
);
#9829=SHAPE_DEFINITION_REPRESENTATION(#9839,#9858);
#9839=PRODUCT_DEFINITION_SHAPE('',$,#9869);
#9858=SHAPE_REPRESENTATION('',(#3488),#9814);
#9866=PRODUCT_DEFINITION_CONTEXT('part definition',#9898,'design');
#9869=PRODUCT_DEFINITION('Hub_01','Hub_01',#9879,#9866);
#9879=PRODUCT_DEFINITION_FORMATION('',$,#9902);
#9898=APPLICATION_CONTEXT(
'Core Data for Automotive Mechanical Design Process');
#9899=PRODUCT_CONTEXT('part definition',#9898,'mechanical');
#9902=PRODUCT('Hub_01','Hub_01',$,(#9899));
#9911=PRESENTATION_STYLE_ASSIGNMENT((#9914));
#9914=SURFACE_STYLE_USAGE(.BOTH.,#9917);
#9917=SURFACE_SIDE_STYLE('',(#9920));
#9920=SURFACE_STYLE_FILL_AREA(#9923);
#9923=FILL_AREA_STYLE('Opaque(78,78,78)',(#9926));
#9926=FILL_AREA_STYLE_COLOUR('Opaque(78,78,78)',#9929);
#9929=COLOUR_RGB('Opaque(78,78,78)', 0.09019608, 0.27058824, 0.51372549);
ENDSEC;
END-ISO-10303-21;
